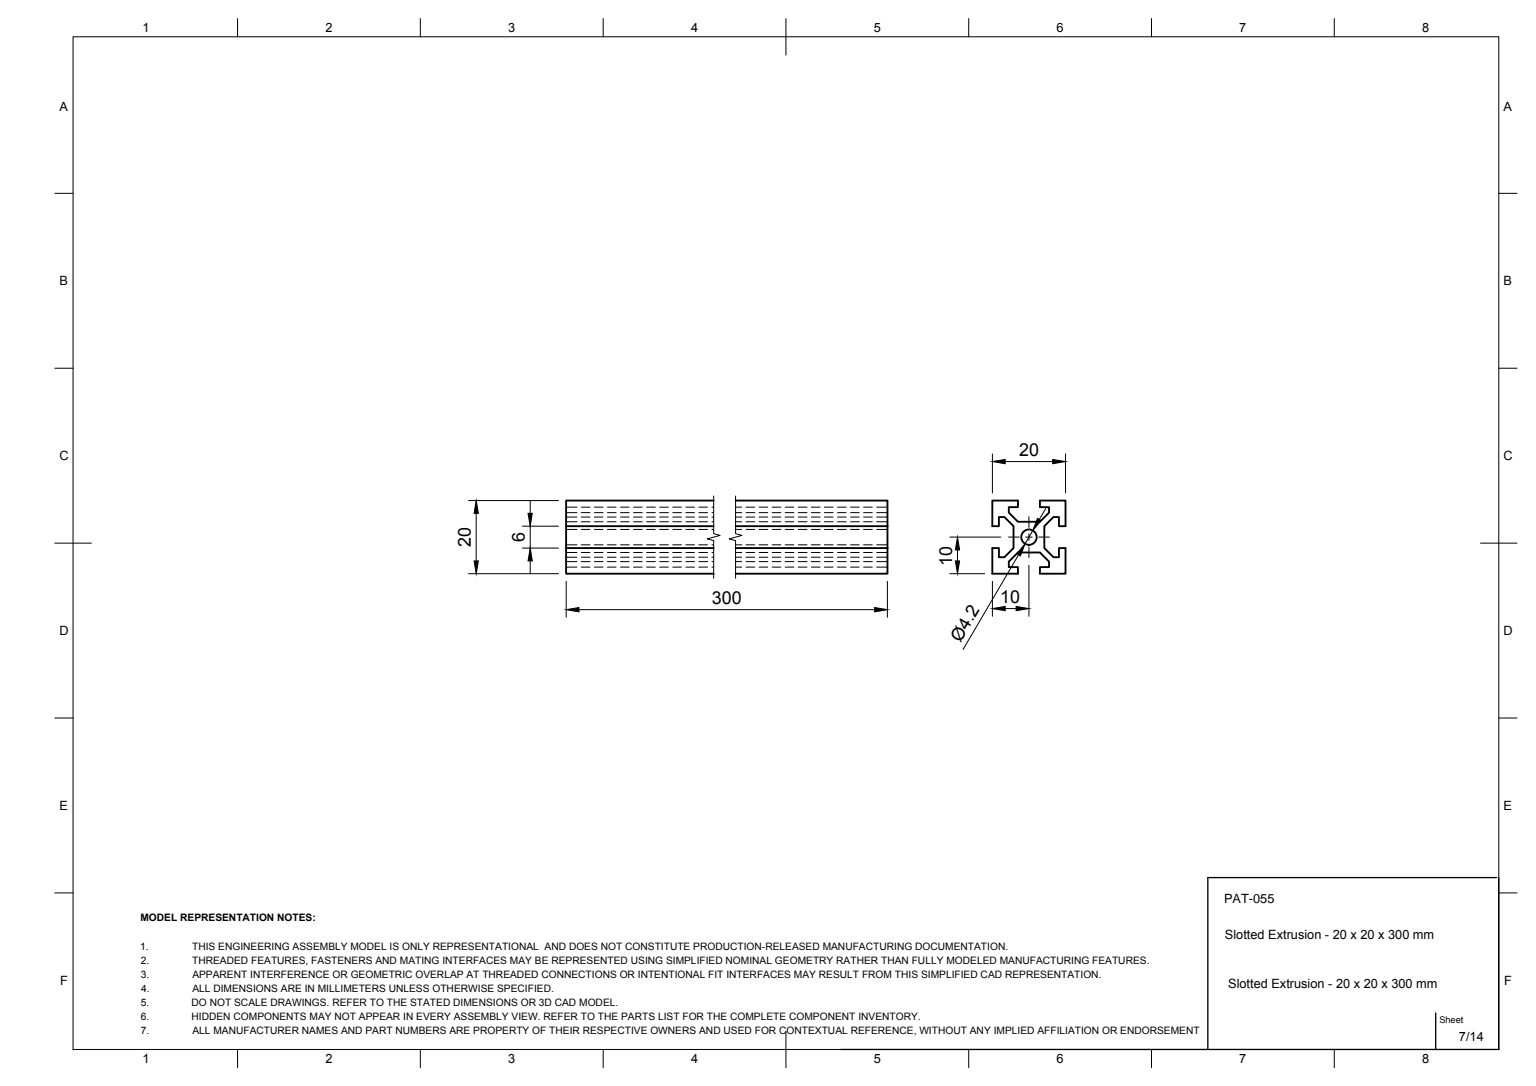
ISO-10303-21;
HEADER;
/* Generated by software containing ST-Developer
 * from STEP Tools, Inc. (www.steptools.com) 
 */

FILE_DESCRIPTION(
/* description */ ('Hinged panel with latch'),
/* implementation_level */ '2;1');

FILE_NAME(
/* name */ 'Slotted Extrusion - 20 x 20 x 300 mm.step',
/* time_stamp */ '2026-10-27T20:36:01-07:00',
/* author */ (''),
/* organization */ (''),
/* preprocessor_version */ 'ST-DEVELOPER v20.2',
/* originating_system */ 'Autodesk Translation Framework v15.17.0.0',
/* authorisation */ '');

FILE_SCHEMA (('AUTOMOTIVE_DESIGN { 1 0 10303 214 3 1 1 }'));
ENDSEC;

DATA;
#10=MECHANICAL_DESIGN_GEOMETRIC_PRESENTATION_REPRESENTATION('',(#297),#6743);
#265=SHAPE_REPRESENTATION_RELATIONSHIP('SRR','None',#6840,#281);
#281=ADVANCED_BREP_SHAPE_REPRESENTATION('',(#313),#6726);
#297=STYLED_ITEM('',(#7017),#313);
#313=MANIFOLD_SOLID_BREP('Body1',#3799);
#329=FACE_BOUND('',#787,.T.);
#330=FACE_BOUND('',#789,.T.);
#378=PLANE('',#4010);
#379=PLANE('',#4011);
#380=PLANE('',#4012);
#381=PLANE('',#4013);
#382=PLANE('',#4014);
#383=PLANE('',#4015);
#384=PLANE('',#4016);
#385=PLANE('',#4017);
#386=PLANE('',#4018);
#387=PLANE('',#4019);
#388=PLANE('',#4020);
#389=PLANE('',#4021);
#390=PLANE('',#4022);
#391=PLANE('',#4023);
#392=PLANE('',#4024);
#393=PLANE('',#4025);
#394=PLANE('',#4026);
#395=PLANE('',#4027);
#396=PLANE('',#4028);
#397=PLANE('',#4029);
#398=PLANE('',#4030);
#399=PLANE('',#4031);
#400=PLANE('',#4032);
#401=PLANE('',#4033);
#402=PLANE('',#4034);
#403=PLANE('',#4035);
#404=PLANE('',#4036);
#405=PLANE('',#4037);
#406=PLANE('',#4038);
#407=PLANE('',#4039);
#408=PLANE('',#4040);
#409=PLANE('',#4041);
#410=PLANE('',#4042);
#411=PLANE('',#4043);
#412=PLANE('',#4044);
#413=PLANE('',#4045);
#414=PLANE('',#4049);
#415=PLANE('',#4050);
#416=PLANE('',#4051);
#417=PLANE('',#4052);
#418=PLANE('',#4053);
#419=PLANE('',#4054);
#420=PLANE('',#4055);
#421=PLANE('',#4056);
#422=PLANE('',#4057);
#423=PLANE('',#4058);
#531=FACE_OUTER_BOUND('',#741,.T.);
#532=FACE_OUTER_BOUND('',#742,.T.);
#533=FACE_OUTER_BOUND('',#743,.T.);
#534=FACE_OUTER_BOUND('',#744,.T.);
#535=FACE_OUTER_BOUND('',#745,.T.);
#536=FACE_OUTER_BOUND('',#746,.T.);
#537=FACE_OUTER_BOUND('',#747,.T.);
#538=FACE_OUTER_BOUND('',#748,.T.);
#539=FACE_OUTER_BOUND('',#749,.T.);
#540=FACE_OUTER_BOUND('',#750,.T.);
#541=FACE_OUTER_BOUND('',#751,.T.);
#542=FACE_OUTER_BOUND('',#752,.T.);
#543=FACE_OUTER_BOUND('',#753,.T.);
#544=FACE_OUTER_BOUND('',#754,.T.);
#545=FACE_OUTER_BOUND('',#755,.T.);
#546=FACE_OUTER_BOUND('',#756,.T.);
#547=FACE_OUTER_BOUND('',#757,.T.);
#548=FACE_OUTER_BOUND('',#758,.T.);
#549=FACE_OUTER_BOUND('',#759,.T.);
#550=FACE_OUTER_BOUND('',#760,.T.);
#551=FACE_OUTER_BOUND('',#761,.T.);
#552=FACE_OUTER_BOUND('',#762,.T.);
#553=FACE_OUTER_BOUND('',#763,.T.);
#554=FACE_OUTER_BOUND('',#764,.T.);
#555=FACE_OUTER_BOUND('',#765,.T.);
#556=FACE_OUTER_BOUND('',#766,.T.);
#557=FACE_OUTER_BOUND('',#767,.T.);
#558=FACE_OUTER_BOUND('',#768,.T.);
#559=FACE_OUTER_BOUND('',#769,.T.);
#560=FACE_OUTER_BOUND('',#770,.T.);
#561=FACE_OUTER_BOUND('',#771,.T.);
#562=FACE_OUTER_BOUND('',#772,.T.);
#563=FACE_OUTER_BOUND('',#773,.T.);
#564=FACE_OUTER_BOUND('',#774,.T.);
#565=FACE_OUTER_BOUND('',#775,.T.);
#566=FACE_OUTER_BOUND('',#776,.T.);
#567=FACE_OUTER_BOUND('',#777,.T.);
#568=FACE_OUTER_BOUND('',#778,.T.);
#569=FACE_OUTER_BOUND('',#779,.T.);
#570=FACE_OUTER_BOUND('',#780,.T.);
#571=FACE_OUTER_BOUND('',#781,.T.);
#572=FACE_OUTER_BOUND('',#782,.T.);
#573=FACE_OUTER_BOUND('',#783,.T.);
#574=FACE_OUTER_BOUND('',#784,.T.);
#575=FACE_OUTER_BOUND('',#785,.T.);
#576=FACE_OUTER_BOUND('',#786,.T.);
#577=FACE_OUTER_BOUND('',#788,.T.);
#741=EDGE_LOOP('',(#2626,#2627,#2628,#2629));
#742=EDGE_LOOP('',(#2630,#2631,#2632,#2633));
#743=EDGE_LOOP('',(#2634,#2635,#2636,#2637));
#744=EDGE_LOOP('',(#2638,#2639,#2640,#2641));
#745=EDGE_LOOP('',(#2642,#2643,#2644,#2645));
#746=EDGE_LOOP('',(#2646,#2647,#2648,#2649));
#747=EDGE_LOOP('',(#2650,#2651,#2652,#2653));
#748=EDGE_LOOP('',(#2654,#2655,#2656,#2657));
#749=EDGE_LOOP('',(#2658,#2659,#2660,#2661));
#750=EDGE_LOOP('',(#2662,#2663,#2664,#2665));
#751=EDGE_LOOP('',(#2666,#2667,#2668,#2669));
#752=EDGE_LOOP('',(#2670,#2671,#2672,#2673));
#753=EDGE_LOOP('',(#2674,#2675,#2676,#2677));
#754=EDGE_LOOP('',(#2678,#2679,#2680,#2681));
#755=EDGE_LOOP('',(#2682,#2683,#2684,#2685));
#756=EDGE_LOOP('',(#2686,#2687,#2688,#2689));
#757=EDGE_LOOP('',(#2690,#2691,#2692,#2693));
#758=EDGE_LOOP('',(#2694,#2695,#2696,#2697));
#759=EDGE_LOOP('',(#2698,#2699,#2700,#2701));
#760=EDGE_LOOP('',(#2702,#2703,#2704,#2705));
#761=EDGE_LOOP('',(#2706,#2707,#2708,#2709));
#762=EDGE_LOOP('',(#2710,#2711,#2712,#2713));
#763=EDGE_LOOP('',(#2714,#2715,#2716,#2717));
#764=EDGE_LOOP('',(#2718,#2719,#2720,#2721));
#765=EDGE_LOOP('',(#2722,#2723,#2724,#2725));
#766=EDGE_LOOP('',(#2726,#2727,#2728,#2729));
#767=EDGE_LOOP('',(#2730,#2731,#2732,#2733));
#768=EDGE_LOOP('',(#2734,#2735,#2736,#2737));
#769=EDGE_LOOP('',(#2738,#2739,#2740,#2741));
#770=EDGE_LOOP('',(#2742,#2743,#2744,#2745));
#771=EDGE_LOOP('',(#2746,#2747,#2748,#2749));
#772=EDGE_LOOP('',(#2750,#2751,#2752,#2753));
#773=EDGE_LOOP('',(#2754,#2755,#2756,#2757));
#774=EDGE_LOOP('',(#2758,#2759,#2760,#2761));
#775=EDGE_LOOP('',(#2762,#2763,#2764,#2765));
#776=EDGE_LOOP('',(#2766,#2767,#2768,#2769));
#777=EDGE_LOOP('',(#2770,#2771,#2772,#2773));
#778=EDGE_LOOP('',(#2774,#2775,#2776,#2777));
#779=EDGE_LOOP('',(#2778,#2779,#2780,#2781));
#780=EDGE_LOOP('',(#2782,#2783,#2784,#2785));
#781=EDGE_LOOP('',(#2786,#2787,#2788,#2789));
#782=EDGE_LOOP('',(#2790,#2791,#2792,#2793));
#783=EDGE_LOOP('',(#2794,#2795,#2796,#2797));
#784=EDGE_LOOP('',(#2798,#2799,#2800,#2801));
#785=EDGE_LOOP('',(#2802,#2803,#2804,#2805));
#786=EDGE_LOOP('',(#2806,#2807,#2808,#2809,#2810,#2811,#2812,#2813,#2814,
#2815,#2816,#2817,#2818,#2819,#2820,#2821,#2822,#2823,#2824,#2825,#2826,
#2827,#2828,#2829,#2830,#2831,#2832,#2833,#2834,#2835,#2836,#2837,#2838,
#2839,#2840,#2841,#2842,#2843,#2844,#2845,#2846,#2847,#2848,#2849));
#787=EDGE_LOOP('',(#2850));
#788=EDGE_LOOP('',(#2851,#2852,#2853,#2854,#2855,#2856,#2857,#2858,#2859,
#2860,#2861,#2862,#2863,#2864,#2865,#2866,#2867,#2868,#2869,#2870,#2871,
#2872,#2873,#2874,#2875,#2876,#2877,#2878,#2879,#2880,#2881,#2882,#2883,
#2884,#2885,#2886,#2887,#2888,#2889,#2890,#2891,#2892,#2893,#2894));
#789=EDGE_LOOP('',(#2895));
#996=LINE('',#5507,#1354);
#997=LINE('',#5509,#1355);
#998=LINE('',#5511,#1356);
#999=LINE('',#5512,#1357);
#1000=LINE('',#5515,#1358);
#1001=LINE('',#5517,#1359);
#1002=LINE('',#5518,#1360);
#1003=LINE('',#5521,#1361);
#1004=LINE('',#5523,#1362);
#1005=LINE('',#5524,#1363);
#1006=LINE('',#5527,#1364);
#1007=LINE('',#5529,#1365);
#1008=LINE('',#5530,#1366);
#1009=LINE('',#5533,#1367);
#1010=LINE('',#5535,#1368);
#1011=LINE('',#5536,#1369);
#1012=LINE('',#5539,#1370);
#1013=LINE('',#5541,#1371);
#1014=LINE('',#5542,#1372);
#1015=LINE('',#5545,#1373);
#1016=LINE('',#5547,#1374);
#1017=LINE('',#5548,#1375);
#1018=LINE('',#5551,#1376);
#1019=LINE('',#5553,#1377);
#1020=LINE('',#5554,#1378);
#1021=LINE('',#5557,#1379);
#1022=LINE('',#5559,#1380);
#1023=LINE('',#5560,#1381);
#1024=LINE('',#5564,#1382);
#1025=LINE('',#5566,#1383);
#1026=LINE('',#5568,#1384);
#1027=LINE('',#5569,#1385);
#1028=LINE('',#5572,#1386);
#1029=LINE('',#5574,#1387);
#1030=LINE('',#5575,#1388);
#1031=LINE('',#5578,#1389);
#1032=LINE('',#5580,#1390);
#1033=LINE('',#5581,#1391);
#1034=LINE('',#5584,#1392);
#1035=LINE('',#5586,#1393);
#1036=LINE('',#5587,#1394);
#1037=LINE('',#5590,#1395);
#1038=LINE('',#5592,#1396);
#1039=LINE('',#5593,#1397);
#1040=LINE('',#5596,#1398);
#1041=LINE('',#5598,#1399);
#1042=LINE('',#5599,#1400);
#1043=LINE('',#5602,#1401);
#1044=LINE('',#5604,#1402);
#1045=LINE('',#5605,#1403);
#1046=LINE('',#5608,#1404);
#1047=LINE('',#5610,#1405);
#1048=LINE('',#5611,#1406);
#1049=LINE('',#5614,#1407);
#1050=LINE('',#5616,#1408);
#1051=LINE('',#5617,#1409);
#1052=LINE('',#5621,#1410);
#1053=LINE('',#5623,#1411);
#1054=LINE('',#5625,#1412);
#1055=LINE('',#5626,#1413);
#1056=LINE('',#5629,#1414);
#1057=LINE('',#5631,#1415);
#1058=LINE('',#5632,#1416);
#1059=LINE('',#5635,#1417);
#1060=LINE('',#5637,#1418);
#1061=LINE('',#5638,#1419);
#1062=LINE('',#5641,#1420);
#1063=LINE('',#5643,#1421);
#1064=LINE('',#5644,#1422);
#1065=LINE('',#5647,#1423);
#1066=LINE('',#5649,#1424);
#1067=LINE('',#5650,#1425);
#1068=LINE('',#5653,#1426);
#1069=LINE('',#5655,#1427);
#1070=LINE('',#5656,#1428);
#1071=LINE('',#5659,#1429);
#1072=LINE('',#5661,#1430);
#1073=LINE('',#5662,#1431);
#1074=LINE('',#5665,#1432);
#1075=LINE('',#5667,#1433);
#1076=LINE('',#5668,#1434);
#1077=LINE('',#5671,#1435);
#1078=LINE('',#5673,#1436);
#1079=LINE('',#5674,#1437);
#1080=LINE('',#5678,#1438);
#1081=LINE('',#5680,#1439);
#1082=LINE('',#5682,#1440);
#1083=LINE('',#5683,#1441);
#1084=LINE('',#5686,#1442);
#1085=LINE('',#5688,#1443);
#1086=LINE('',#5689,#1444);
#1087=LINE('',#5692,#1445);
#1088=LINE('',#5694,#1446);
#1089=LINE('',#5695,#1447);
#1090=LINE('',#5698,#1448);
#1091=LINE('',#5700,#1449);
#1092=LINE('',#5701,#1450);
#1093=LINE('',#5704,#1451);
#1094=LINE('',#5706,#1452);
#1095=LINE('',#5707,#1453);
#1096=LINE('',#5710,#1454);
#1097=LINE('',#5712,#1455);
#1098=LINE('',#5713,#1456);
#1099=LINE('',#5716,#1457);
#1100=LINE('',#5718,#1458);
#1101=LINE('',#5719,#1459);
#1102=LINE('',#5722,#1460);
#1103=LINE('',#5724,#1461);
#1104=LINE('',#5725,#1462);
#1105=LINE('',#5728,#1463);
#1106=LINE('',#5730,#1464);
#1107=LINE('',#5731,#1465);
#1108=LINE('',#5736,#1466);
#1109=LINE('',#5740,#1467);
#1110=LINE('',#5742,#1468);
#1111=LINE('',#5743,#1469);
#1112=LINE('',#5746,#1470);
#1113=LINE('',#5748,#1471);
#1114=LINE('',#5749,#1472);
#1115=LINE('',#5751,#1473);
#1116=LINE('',#5752,#1474);
#1117=LINE('',#5755,#1475);
#1118=LINE('',#5757,#1476);
#1119=LINE('',#5758,#1477);
#1120=LINE('',#5760,#1478);
#1121=LINE('',#5761,#1479);
#1122=LINE('',#5764,#1480);
#1123=LINE('',#5766,#1481);
#1124=LINE('',#5767,#1482);
#1125=LINE('',#5769,#1483);
#1126=LINE('',#5770,#1484);
#1127=LINE('',#5772,#1485);
#1128=LINE('',#5773,#1486);
#1354=VECTOR('',#4412,1.);
#1355=VECTOR('',#4413,1.);
#1356=VECTOR('',#4414,1.);
#1357=VECTOR('',#4415,1.);
#1358=VECTOR('',#4418,1.);
#1359=VECTOR('',#4419,1.);
#1360=VECTOR('',#4420,1.);
#1361=VECTOR('',#4423,1.);
#1362=VECTOR('',#4424,1.);
#1363=VECTOR('',#4425,1.);
#1364=VECTOR('',#4428,1.);
#1365=VECTOR('',#4429,1.);
#1366=VECTOR('',#4430,1.);
#1367=VECTOR('',#4433,1.);
#1368=VECTOR('',#4434,1.);
#1369=VECTOR('',#4435,1.);
#1370=VECTOR('',#4438,1.);
#1371=VECTOR('',#4439,1.);
#1372=VECTOR('',#4440,1.);
#1373=VECTOR('',#4443,1.);
#1374=VECTOR('',#4444,1.);
#1375=VECTOR('',#4445,1.);
#1376=VECTOR('',#4448,1.);
#1377=VECTOR('',#4449,1.);
#1378=VECTOR('',#4450,1.);
#1379=VECTOR('',#4453,1.);
#1380=VECTOR('',#4454,1.);
#1381=VECTOR('',#4455,1.);
#1382=VECTOR('',#4458,1.);
#1383=VECTOR('',#4459,1.);
#1384=VECTOR('',#4460,1.);
#1385=VECTOR('',#4461,1.);
#1386=VECTOR('',#4464,1.);
#1387=VECTOR('',#4465,1.);
#1388=VECTOR('',#4466,1.);
#1389=VECTOR('',#4469,1.);
#1390=VECTOR('',#4470,1.);
#1391=VECTOR('',#4471,1.);
#1392=VECTOR('',#4474,1.);
#1393=VECTOR('',#4475,1.);
#1394=VECTOR('',#4476,1.);
#1395=VECTOR('',#4479,1.);
#1396=VECTOR('',#4480,1.);
#1397=VECTOR('',#4481,1.);
#1398=VECTOR('',#4484,1.);
#1399=VECTOR('',#4485,1.);
#1400=VECTOR('',#4486,1.);
#1401=VECTOR('',#4489,1.);
#1402=VECTOR('',#4490,1.);
#1403=VECTOR('',#4491,1.);
#1404=VECTOR('',#4494,1.);
#1405=VECTOR('',#4495,1.);
#1406=VECTOR('',#4496,1.);
#1407=VECTOR('',#4499,1.);
#1408=VECTOR('',#4500,1.);
#1409=VECTOR('',#4501,1.);
#1410=VECTOR('',#4504,1.);
#1411=VECTOR('',#4505,1.);
#1412=VECTOR('',#4506,1.);
#1413=VECTOR('',#4507,1.);
#1414=VECTOR('',#4510,1.);
#1415=VECTOR('',#4511,1.);
#1416=VECTOR('',#4512,1.);
#1417=VECTOR('',#4515,1.);
#1418=VECTOR('',#4516,1.);
#1419=VECTOR('',#4517,1.);
#1420=VECTOR('',#4520,1.);
#1421=VECTOR('',#4521,1.);
#1422=VECTOR('',#4522,1.);
#1423=VECTOR('',#4525,1.);
#1424=VECTOR('',#4526,1.);
#1425=VECTOR('',#4527,1.);
#1426=VECTOR('',#4530,1.);
#1427=VECTOR('',#4531,1.);
#1428=VECTOR('',#4532,1.);
#1429=VECTOR('',#4535,1.);
#1430=VECTOR('',#4536,1.);
#1431=VECTOR('',#4537,1.);
#1432=VECTOR('',#4540,1.);
#1433=VECTOR('',#4541,1.);
#1434=VECTOR('',#4542,1.);
#1435=VECTOR('',#4545,1.);
#1436=VECTOR('',#4546,1.);
#1437=VECTOR('',#4547,1.);
#1438=VECTOR('',#4550,1.);
#1439=VECTOR('',#4551,1.);
#1440=VECTOR('',#4552,1.);
#1441=VECTOR('',#4553,1.);
#1442=VECTOR('',#4556,1.);
#1443=VECTOR('',#4557,1.);
#1444=VECTOR('',#4558,1.);
#1445=VECTOR('',#4561,1.);
#1446=VECTOR('',#4562,1.);
#1447=VECTOR('',#4563,1.);
#1448=VECTOR('',#4566,1.);
#1449=VECTOR('',#4567,1.);
#1450=VECTOR('',#4568,1.);
#1451=VECTOR('',#4571,1.);
#1452=VECTOR('',#4572,1.);
#1453=VECTOR('',#4573,1.);
#1454=VECTOR('',#4576,1.);
#1455=VECTOR('',#4577,1.);
#1456=VECTOR('',#4578,1.);
#1457=VECTOR('',#4581,1.);
#1458=VECTOR('',#4582,1.);
#1459=VECTOR('',#4583,1.);
#1460=VECTOR('',#4586,1.);
#1461=VECTOR('',#4587,1.);
#1462=VECTOR('',#4588,1.);
#1463=VECTOR('',#4591,1.);
#1464=VECTOR('',#4592,1.);
#1465=VECTOR('',#4593,1.);
#1466=VECTOR('',#4598,0.21);
#1467=VECTOR('',#4603,1.);
#1468=VECTOR('',#4604,1.);
#1469=VECTOR('',#4605,1.);
#1470=VECTOR('',#4608,1.);
#1471=VECTOR('',#4609,1.);
#1472=VECTOR('',#4610,1.);
#1473=VECTOR('',#4613,1.);
#1474=VECTOR('',#4614,1.);
#1475=VECTOR('',#4617,1.);
#1476=VECTOR('',#4618,1.);
#1477=VECTOR('',#4619,1.);
#1478=VECTOR('',#4622,1.);
#1479=VECTOR('',#4623,1.);
#1480=VECTOR('',#4626,1.);
#1481=VECTOR('',#4627,1.);
#1482=VECTOR('',#4628,1.);
#1483=VECTOR('',#4631,1.);
#1484=VECTOR('',#4632,1.);
#1485=VECTOR('',#4635,1.);
#1486=VECTOR('',#4636,1.);
#1702=CIRCLE('',#4047,0.21);
#1703=CIRCLE('',#4048,0.21);
#1803=VERTEX_POINT('',#5505);
#1804=VERTEX_POINT('',#5506);
#1805=VERTEX_POINT('',#5508);
#1806=VERTEX_POINT('',#5510);
#1807=VERTEX_POINT('',#5514);
#1808=VERTEX_POINT('',#5516);
#1809=VERTEX_POINT('',#5520);
#1810=VERTEX_POINT('',#5522);
#1811=VERTEX_POINT('',#5526);
#1812=VERTEX_POINT('',#5528);
#1813=VERTEX_POINT('',#5532);
#1814=VERTEX_POINT('',#5534);
#1815=VERTEX_POINT('',#5538);
#1816=VERTEX_POINT('',#5540);
#1817=VERTEX_POINT('',#5544);
#1818=VERTEX_POINT('',#5546);
#1819=VERTEX_POINT('',#5550);
#1820=VERTEX_POINT('',#5552);
#1821=VERTEX_POINT('',#5556);
#1822=VERTEX_POINT('',#5558);
#1823=VERTEX_POINT('',#5562);
#1824=VERTEX_POINT('',#5563);
#1825=VERTEX_POINT('',#5565);
#1826=VERTEX_POINT('',#5567);
#1827=VERTEX_POINT('',#5571);
#1828=VERTEX_POINT('',#5573);
#1829=VERTEX_POINT('',#5577);
#1830=VERTEX_POINT('',#5579);
#1831=VERTEX_POINT('',#5583);
#1832=VERTEX_POINT('',#5585);
#1833=VERTEX_POINT('',#5589);
#1834=VERTEX_POINT('',#5591);
#1835=VERTEX_POINT('',#5595);
#1836=VERTEX_POINT('',#5597);
#1837=VERTEX_POINT('',#5601);
#1838=VERTEX_POINT('',#5603);
#1839=VERTEX_POINT('',#5607);
#1840=VERTEX_POINT('',#5609);
#1841=VERTEX_POINT('',#5613);
#1842=VERTEX_POINT('',#5615);
#1843=VERTEX_POINT('',#5619);
#1844=VERTEX_POINT('',#5620);
#1845=VERTEX_POINT('',#5622);
#1846=VERTEX_POINT('',#5624);
#1847=VERTEX_POINT('',#5628);
#1848=VERTEX_POINT('',#5630);
#1849=VERTEX_POINT('',#5634);
#1850=VERTEX_POINT('',#5636);
#1851=VERTEX_POINT('',#5640);
#1852=VERTEX_POINT('',#5642);
#1853=VERTEX_POINT('',#5646);
#1854=VERTEX_POINT('',#5648);
#1855=VERTEX_POINT('',#5652);
#1856=VERTEX_POINT('',#5654);
#1857=VERTEX_POINT('',#5658);
#1858=VERTEX_POINT('',#5660);
#1859=VERTEX_POINT('',#5664);
#1860=VERTEX_POINT('',#5666);
#1861=VERTEX_POINT('',#5670);
#1862=VERTEX_POINT('',#5672);
#1863=VERTEX_POINT('',#5676);
#1864=VERTEX_POINT('',#5677);
#1865=VERTEX_POINT('',#5679);
#1866=VERTEX_POINT('',#5681);
#1867=VERTEX_POINT('',#5685);
#1868=VERTEX_POINT('',#5687);
#1869=VERTEX_POINT('',#5691);
#1870=VERTEX_POINT('',#5693);
#1871=VERTEX_POINT('',#5697);
#1872=VERTEX_POINT('',#5699);
#1873=VERTEX_POINT('',#5703);
#1874=VERTEX_POINT('',#5705);
#1875=VERTEX_POINT('',#5709);
#1876=VERTEX_POINT('',#5711);
#1877=VERTEX_POINT('',#5715);
#1878=VERTEX_POINT('',#5717);
#1879=VERTEX_POINT('',#5721);
#1880=VERTEX_POINT('',#5723);
#1881=VERTEX_POINT('',#5727);
#1882=VERTEX_POINT('',#5729);
#1883=VERTEX_POINT('',#5733);
#1884=VERTEX_POINT('',#5735);
#1885=VERTEX_POINT('',#5739);
#1886=VERTEX_POINT('',#5741);
#1887=VERTEX_POINT('',#5745);
#1888=VERTEX_POINT('',#5747);
#1889=VERTEX_POINT('',#5754);
#1890=VERTEX_POINT('',#5756);
#1891=VERTEX_POINT('',#5763);
#1892=VERTEX_POINT('',#5765);
#2125=EDGE_CURVE('',#1803,#1804,#996,.T.);
#2126=EDGE_CURVE('',#1803,#1805,#997,.T.);
#2127=EDGE_CURVE('',#1806,#1805,#998,.T.);
#2128=EDGE_CURVE('',#1804,#1806,#999,.T.);
#2129=EDGE_CURVE('',#1807,#1803,#1000,.T.);
#2130=EDGE_CURVE('',#1807,#1808,#1001,.T.);
#2131=EDGE_CURVE('',#1805,#1808,#1002,.T.);
#2132=EDGE_CURVE('',#1809,#1807,#1003,.T.);
#2133=EDGE_CURVE('',#1809,#1810,#1004,.T.);
#2134=EDGE_CURVE('',#1808,#1810,#1005,.T.);
#2135=EDGE_CURVE('',#1811,#1809,#1006,.T.);
#2136=EDGE_CURVE('',#1811,#1812,#1007,.T.);
#2137=EDGE_CURVE('',#1810,#1812,#1008,.T.);
#2138=EDGE_CURVE('',#1813,#1811,#1009,.T.);
#2139=EDGE_CURVE('',#1813,#1814,#1010,.T.);
#2140=EDGE_CURVE('',#1812,#1814,#1011,.T.);
#2141=EDGE_CURVE('',#1815,#1813,#1012,.T.);
#2142=EDGE_CURVE('',#1815,#1816,#1013,.T.);
#2143=EDGE_CURVE('',#1814,#1816,#1014,.T.);
#2144=EDGE_CURVE('',#1817,#1815,#1015,.T.);
#2145=EDGE_CURVE('',#1817,#1818,#1016,.T.);
#2146=EDGE_CURVE('',#1816,#1818,#1017,.T.);
#2147=EDGE_CURVE('',#1819,#1817,#1018,.T.);
#2148=EDGE_CURVE('',#1819,#1820,#1019,.T.);
#2149=EDGE_CURVE('',#1818,#1820,#1020,.T.);
#2150=EDGE_CURVE('',#1821,#1819,#1021,.T.);
#2151=EDGE_CURVE('',#1822,#1821,#1022,.T.);
#2152=EDGE_CURVE('',#1820,#1822,#1023,.T.);
#2153=EDGE_CURVE('',#1823,#1824,#1024,.T.);
#2154=EDGE_CURVE('',#1823,#1825,#1025,.T.);
#2155=EDGE_CURVE('',#1826,#1825,#1026,.T.);
#2156=EDGE_CURVE('',#1824,#1826,#1027,.T.);
#2157=EDGE_CURVE('',#1827,#1823,#1028,.T.);
#2158=EDGE_CURVE('',#1827,#1828,#1029,.T.);
#2159=EDGE_CURVE('',#1825,#1828,#1030,.T.);
#2160=EDGE_CURVE('',#1829,#1827,#1031,.T.);
#2161=EDGE_CURVE('',#1829,#1830,#1032,.T.);
#2162=EDGE_CURVE('',#1828,#1830,#1033,.T.);
#2163=EDGE_CURVE('',#1831,#1829,#1034,.T.);
#2164=EDGE_CURVE('',#1831,#1832,#1035,.T.);
#2165=EDGE_CURVE('',#1830,#1832,#1036,.T.);
#2166=EDGE_CURVE('',#1833,#1831,#1037,.T.);
#2167=EDGE_CURVE('',#1833,#1834,#1038,.T.);
#2168=EDGE_CURVE('',#1832,#1834,#1039,.T.);
#2169=EDGE_CURVE('',#1835,#1833,#1040,.T.);
#2170=EDGE_CURVE('',#1835,#1836,#1041,.T.);
#2171=EDGE_CURVE('',#1834,#1836,#1042,.T.);
#2172=EDGE_CURVE('',#1837,#1835,#1043,.T.);
#2173=EDGE_CURVE('',#1837,#1838,#1044,.T.);
#2174=EDGE_CURVE('',#1836,#1838,#1045,.T.);
#2175=EDGE_CURVE('',#1839,#1837,#1046,.T.);
#2176=EDGE_CURVE('',#1839,#1840,#1047,.T.);
#2177=EDGE_CURVE('',#1838,#1840,#1048,.T.);
#2178=EDGE_CURVE('',#1841,#1839,#1049,.T.);
#2179=EDGE_CURVE('',#1842,#1841,#1050,.T.);
#2180=EDGE_CURVE('',#1840,#1842,#1051,.T.);
#2181=EDGE_CURVE('',#1843,#1844,#1052,.T.);
#2182=EDGE_CURVE('',#1843,#1845,#1053,.T.);
#2183=EDGE_CURVE('',#1846,#1845,#1054,.T.);
#2184=EDGE_CURVE('',#1844,#1846,#1055,.T.);
#2185=EDGE_CURVE('',#1847,#1843,#1056,.T.);
#2186=EDGE_CURVE('',#1847,#1848,#1057,.T.);
#2187=EDGE_CURVE('',#1845,#1848,#1058,.T.);
#2188=EDGE_CURVE('',#1849,#1847,#1059,.T.);
#2189=EDGE_CURVE('',#1849,#1850,#1060,.T.);
#2190=EDGE_CURVE('',#1848,#1850,#1061,.T.);
#2191=EDGE_CURVE('',#1851,#1849,#1062,.T.);
#2192=EDGE_CURVE('',#1851,#1852,#1063,.T.);
#2193=EDGE_CURVE('',#1850,#1852,#1064,.T.);
#2194=EDGE_CURVE('',#1853,#1851,#1065,.T.);
#2195=EDGE_CURVE('',#1853,#1854,#1066,.T.);
#2196=EDGE_CURVE('',#1852,#1854,#1067,.T.);
#2197=EDGE_CURVE('',#1855,#1853,#1068,.T.);
#2198=EDGE_CURVE('',#1855,#1856,#1069,.T.);
#2199=EDGE_CURVE('',#1854,#1856,#1070,.T.);
#2200=EDGE_CURVE('',#1857,#1855,#1071,.T.);
#2201=EDGE_CURVE('',#1857,#1858,#1072,.T.);
#2202=EDGE_CURVE('',#1856,#1858,#1073,.T.);
#2203=EDGE_CURVE('',#1859,#1857,#1074,.T.);
#2204=EDGE_CURVE('',#1859,#1860,#1075,.T.);
#2205=EDGE_CURVE('',#1858,#1860,#1076,.T.);
#2206=EDGE_CURVE('',#1861,#1859,#1077,.T.);
#2207=EDGE_CURVE('',#1862,#1861,#1078,.T.);
#2208=EDGE_CURVE('',#1860,#1862,#1079,.T.);
#2209=EDGE_CURVE('',#1863,#1864,#1080,.T.);
#2210=EDGE_CURVE('',#1863,#1865,#1081,.T.);
#2211=EDGE_CURVE('',#1866,#1865,#1082,.T.);
#2212=EDGE_CURVE('',#1864,#1866,#1083,.T.);
#2213=EDGE_CURVE('',#1867,#1863,#1084,.T.);
#2214=EDGE_CURVE('',#1867,#1868,#1085,.T.);
#2215=EDGE_CURVE('',#1865,#1868,#1086,.T.);
#2216=EDGE_CURVE('',#1869,#1867,#1087,.T.);
#2217=EDGE_CURVE('',#1869,#1870,#1088,.T.);
#2218=EDGE_CURVE('',#1868,#1870,#1089,.T.);
#2219=EDGE_CURVE('',#1871,#1869,#1090,.T.);
#2220=EDGE_CURVE('',#1871,#1872,#1091,.T.);
#2221=EDGE_CURVE('',#1870,#1872,#1092,.T.);
#2222=EDGE_CURVE('',#1873,#1871,#1093,.T.);
#2223=EDGE_CURVE('',#1873,#1874,#1094,.T.);
#2224=EDGE_CURVE('',#1872,#1874,#1095,.T.);
#2225=EDGE_CURVE('',#1875,#1873,#1096,.T.);
#2226=EDGE_CURVE('',#1875,#1876,#1097,.T.);
#2227=EDGE_CURVE('',#1874,#1876,#1098,.T.);
#2228=EDGE_CURVE('',#1877,#1875,#1099,.T.);
#2229=EDGE_CURVE('',#1877,#1878,#1100,.T.);
#2230=EDGE_CURVE('',#1876,#1878,#1101,.T.);
#2231=EDGE_CURVE('',#1879,#1877,#1102,.T.);
#2232=EDGE_CURVE('',#1879,#1880,#1103,.T.);
#2233=EDGE_CURVE('',#1878,#1880,#1104,.T.);
#2234=EDGE_CURVE('',#1881,#1879,#1105,.T.);
#2235=EDGE_CURVE('',#1882,#1881,#1106,.T.);
#2236=EDGE_CURVE('',#1880,#1882,#1107,.T.);
#2237=EDGE_CURVE('',#1883,#1883,#1702,.T.);
#2238=EDGE_CURVE('',#1883,#1884,#1108,.T.);
#2239=EDGE_CURVE('',#1884,#1884,#1703,.T.);
#2240=EDGE_CURVE('',#1821,#1885,#1109,.T.);
#2241=EDGE_CURVE('',#1885,#1886,#1110,.T.);
#2242=EDGE_CURVE('',#1822,#1886,#1111,.T.);
#2243=EDGE_CURVE('',#1887,#1806,#1112,.T.);
#2244=EDGE_CURVE('',#1888,#1887,#1113,.T.);
#2245=EDGE_CURVE('',#1888,#1804,#1114,.T.);
#2246=EDGE_CURVE('',#1841,#1888,#1115,.T.);
#2247=EDGE_CURVE('',#1842,#1887,#1116,.T.);
#2248=EDGE_CURVE('',#1889,#1826,#1117,.T.);
#2249=EDGE_CURVE('',#1890,#1889,#1118,.T.);
#2250=EDGE_CURVE('',#1890,#1824,#1119,.T.);
#2251=EDGE_CURVE('',#1861,#1890,#1120,.T.);
#2252=EDGE_CURVE('',#1862,#1889,#1121,.T.);
#2253=EDGE_CURVE('',#1891,#1846,#1122,.T.);
#2254=EDGE_CURVE('',#1892,#1891,#1123,.T.);
#2255=EDGE_CURVE('',#1892,#1844,#1124,.T.);
#2256=EDGE_CURVE('',#1881,#1892,#1125,.T.);
#2257=EDGE_CURVE('',#1882,#1891,#1126,.T.);
#2258=EDGE_CURVE('',#1886,#1866,#1127,.T.);
#2259=EDGE_CURVE('',#1885,#1864,#1128,.T.);
#2626=ORIENTED_EDGE('',*,*,#2125,.F.);
#2627=ORIENTED_EDGE('',*,*,#2126,.T.);
#2628=ORIENTED_EDGE('',*,*,#2127,.F.);
#2629=ORIENTED_EDGE('',*,*,#2128,.F.);
#2630=ORIENTED_EDGE('',*,*,#2129,.F.);
#2631=ORIENTED_EDGE('',*,*,#2130,.T.);
#2632=ORIENTED_EDGE('',*,*,#2131,.F.);
#2633=ORIENTED_EDGE('',*,*,#2126,.F.);
#2634=ORIENTED_EDGE('',*,*,#2132,.F.);
#2635=ORIENTED_EDGE('',*,*,#2133,.T.);
#2636=ORIENTED_EDGE('',*,*,#2134,.F.);
#2637=ORIENTED_EDGE('',*,*,#2130,.F.);
#2638=ORIENTED_EDGE('',*,*,#2135,.F.);
#2639=ORIENTED_EDGE('',*,*,#2136,.T.);
#2640=ORIENTED_EDGE('',*,*,#2137,.F.);
#2641=ORIENTED_EDGE('',*,*,#2133,.F.);
#2642=ORIENTED_EDGE('',*,*,#2138,.F.);
#2643=ORIENTED_EDGE('',*,*,#2139,.T.);
#2644=ORIENTED_EDGE('',*,*,#2140,.F.);
#2645=ORIENTED_EDGE('',*,*,#2136,.F.);
#2646=ORIENTED_EDGE('',*,*,#2141,.F.);
#2647=ORIENTED_EDGE('',*,*,#2142,.T.);
#2648=ORIENTED_EDGE('',*,*,#2143,.F.);
#2649=ORIENTED_EDGE('',*,*,#2139,.F.);
#2650=ORIENTED_EDGE('',*,*,#2144,.F.);
#2651=ORIENTED_EDGE('',*,*,#2145,.T.);
#2652=ORIENTED_EDGE('',*,*,#2146,.F.);
#2653=ORIENTED_EDGE('',*,*,#2142,.F.);
#2654=ORIENTED_EDGE('',*,*,#2147,.F.);
#2655=ORIENTED_EDGE('',*,*,#2148,.T.);
#2656=ORIENTED_EDGE('',*,*,#2149,.F.);
#2657=ORIENTED_EDGE('',*,*,#2145,.F.);
#2658=ORIENTED_EDGE('',*,*,#2150,.F.);
#2659=ORIENTED_EDGE('',*,*,#2151,.F.);
#2660=ORIENTED_EDGE('',*,*,#2152,.F.);
#2661=ORIENTED_EDGE('',*,*,#2148,.F.);
#2662=ORIENTED_EDGE('',*,*,#2153,.F.);
#2663=ORIENTED_EDGE('',*,*,#2154,.T.);
#2664=ORIENTED_EDGE('',*,*,#2155,.F.);
#2665=ORIENTED_EDGE('',*,*,#2156,.F.);
#2666=ORIENTED_EDGE('',*,*,#2157,.F.);
#2667=ORIENTED_EDGE('',*,*,#2158,.T.);
#2668=ORIENTED_EDGE('',*,*,#2159,.F.);
#2669=ORIENTED_EDGE('',*,*,#2154,.F.);
#2670=ORIENTED_EDGE('',*,*,#2160,.F.);
#2671=ORIENTED_EDGE('',*,*,#2161,.T.);
#2672=ORIENTED_EDGE('',*,*,#2162,.F.);
#2673=ORIENTED_EDGE('',*,*,#2158,.F.);
#2674=ORIENTED_EDGE('',*,*,#2163,.F.);
#2675=ORIENTED_EDGE('',*,*,#2164,.T.);
#2676=ORIENTED_EDGE('',*,*,#2165,.F.);
#2677=ORIENTED_EDGE('',*,*,#2161,.F.);
#2678=ORIENTED_EDGE('',*,*,#2166,.F.);
#2679=ORIENTED_EDGE('',*,*,#2167,.T.);
#2680=ORIENTED_EDGE('',*,*,#2168,.F.);
#2681=ORIENTED_EDGE('',*,*,#2164,.F.);
#2682=ORIENTED_EDGE('',*,*,#2169,.F.);
#2683=ORIENTED_EDGE('',*,*,#2170,.T.);
#2684=ORIENTED_EDGE('',*,*,#2171,.F.);
#2685=ORIENTED_EDGE('',*,*,#2167,.F.);
#2686=ORIENTED_EDGE('',*,*,#2172,.F.);
#2687=ORIENTED_EDGE('',*,*,#2173,.T.);
#2688=ORIENTED_EDGE('',*,*,#2174,.F.);
#2689=ORIENTED_EDGE('',*,*,#2170,.F.);
#2690=ORIENTED_EDGE('',*,*,#2175,.F.);
#2691=ORIENTED_EDGE('',*,*,#2176,.T.);
#2692=ORIENTED_EDGE('',*,*,#2177,.F.);
#2693=ORIENTED_EDGE('',*,*,#2173,.F.);
#2694=ORIENTED_EDGE('',*,*,#2178,.F.);
#2695=ORIENTED_EDGE('',*,*,#2179,.F.);
#2696=ORIENTED_EDGE('',*,*,#2180,.F.);
#2697=ORIENTED_EDGE('',*,*,#2176,.F.);
#2698=ORIENTED_EDGE('',*,*,#2181,.F.);
#2699=ORIENTED_EDGE('',*,*,#2182,.T.);
#2700=ORIENTED_EDGE('',*,*,#2183,.F.);
#2701=ORIENTED_EDGE('',*,*,#2184,.F.);
#2702=ORIENTED_EDGE('',*,*,#2185,.F.);
#2703=ORIENTED_EDGE('',*,*,#2186,.T.);
#2704=ORIENTED_EDGE('',*,*,#2187,.F.);
#2705=ORIENTED_EDGE('',*,*,#2182,.F.);
#2706=ORIENTED_EDGE('',*,*,#2188,.F.);
#2707=ORIENTED_EDGE('',*,*,#2189,.T.);
#2708=ORIENTED_EDGE('',*,*,#2190,.F.);
#2709=ORIENTED_EDGE('',*,*,#2186,.F.);
#2710=ORIENTED_EDGE('',*,*,#2191,.F.);
#2711=ORIENTED_EDGE('',*,*,#2192,.T.);
#2712=ORIENTED_EDGE('',*,*,#2193,.F.);
#2713=ORIENTED_EDGE('',*,*,#2189,.F.);
#2714=ORIENTED_EDGE('',*,*,#2194,.F.);
#2715=ORIENTED_EDGE('',*,*,#2195,.T.);
#2716=ORIENTED_EDGE('',*,*,#2196,.F.);
#2717=ORIENTED_EDGE('',*,*,#2192,.F.);
#2718=ORIENTED_EDGE('',*,*,#2197,.F.);
#2719=ORIENTED_EDGE('',*,*,#2198,.T.);
#2720=ORIENTED_EDGE('',*,*,#2199,.F.);
#2721=ORIENTED_EDGE('',*,*,#2195,.F.);
#2722=ORIENTED_EDGE('',*,*,#2200,.F.);
#2723=ORIENTED_EDGE('',*,*,#2201,.T.);
#2724=ORIENTED_EDGE('',*,*,#2202,.F.);
#2725=ORIENTED_EDGE('',*,*,#2198,.F.);
#2726=ORIENTED_EDGE('',*,*,#2203,.F.);
#2727=ORIENTED_EDGE('',*,*,#2204,.T.);
#2728=ORIENTED_EDGE('',*,*,#2205,.F.);
#2729=ORIENTED_EDGE('',*,*,#2201,.F.);
#2730=ORIENTED_EDGE('',*,*,#2206,.F.);
#2731=ORIENTED_EDGE('',*,*,#2207,.F.);
#2732=ORIENTED_EDGE('',*,*,#2208,.F.);
#2733=ORIENTED_EDGE('',*,*,#2204,.F.);
#2734=ORIENTED_EDGE('',*,*,#2209,.F.);
#2735=ORIENTED_EDGE('',*,*,#2210,.T.);
#2736=ORIENTED_EDGE('',*,*,#2211,.F.);
#2737=ORIENTED_EDGE('',*,*,#2212,.F.);
#2738=ORIENTED_EDGE('',*,*,#2213,.F.);
#2739=ORIENTED_EDGE('',*,*,#2214,.T.);
#2740=ORIENTED_EDGE('',*,*,#2215,.F.);
#2741=ORIENTED_EDGE('',*,*,#2210,.F.);
#2742=ORIENTED_EDGE('',*,*,#2216,.F.);
#2743=ORIENTED_EDGE('',*,*,#2217,.T.);
#2744=ORIENTED_EDGE('',*,*,#2218,.F.);
#2745=ORIENTED_EDGE('',*,*,#2214,.F.);
#2746=ORIENTED_EDGE('',*,*,#2219,.F.);
#2747=ORIENTED_EDGE('',*,*,#2220,.T.);
#2748=ORIENTED_EDGE('',*,*,#2221,.F.);
#2749=ORIENTED_EDGE('',*,*,#2217,.F.);
#2750=ORIENTED_EDGE('',*,*,#2222,.F.);
#2751=ORIENTED_EDGE('',*,*,#2223,.T.);
#2752=ORIENTED_EDGE('',*,*,#2224,.F.);
#2753=ORIENTED_EDGE('',*,*,#2220,.F.);
#2754=ORIENTED_EDGE('',*,*,#2225,.F.);
#2755=ORIENTED_EDGE('',*,*,#2226,.T.);
#2756=ORIENTED_EDGE('',*,*,#2227,.F.);
#2757=ORIENTED_EDGE('',*,*,#2223,.F.);
#2758=ORIENTED_EDGE('',*,*,#2228,.F.);
#2759=ORIENTED_EDGE('',*,*,#2229,.T.);
#2760=ORIENTED_EDGE('',*,*,#2230,.F.);
#2761=ORIENTED_EDGE('',*,*,#2226,.F.);
#2762=ORIENTED_EDGE('',*,*,#2231,.F.);
#2763=ORIENTED_EDGE('',*,*,#2232,.T.);
#2764=ORIENTED_EDGE('',*,*,#2233,.F.);
#2765=ORIENTED_EDGE('',*,*,#2229,.F.);
#2766=ORIENTED_EDGE('',*,*,#2234,.F.);
#2767=ORIENTED_EDGE('',*,*,#2235,.F.);
#2768=ORIENTED_EDGE('',*,*,#2236,.F.);
#2769=ORIENTED_EDGE('',*,*,#2232,.F.);
#2770=ORIENTED_EDGE('',*,*,#2237,.F.);
#2771=ORIENTED_EDGE('',*,*,#2238,.T.);
#2772=ORIENTED_EDGE('',*,*,#2239,.F.);
#2773=ORIENTED_EDGE('',*,*,#2238,.F.);
#2774=ORIENTED_EDGE('',*,*,#2151,.T.);
#2775=ORIENTED_EDGE('',*,*,#2240,.T.);
#2776=ORIENTED_EDGE('',*,*,#2241,.T.);
#2777=ORIENTED_EDGE('',*,*,#2242,.F.);
#2778=ORIENTED_EDGE('',*,*,#2128,.T.);
#2779=ORIENTED_EDGE('',*,*,#2243,.F.);
#2780=ORIENTED_EDGE('',*,*,#2244,.F.);
#2781=ORIENTED_EDGE('',*,*,#2245,.T.);
#2782=ORIENTED_EDGE('',*,*,#2179,.T.);
#2783=ORIENTED_EDGE('',*,*,#2246,.T.);
#2784=ORIENTED_EDGE('',*,*,#2244,.T.);
#2785=ORIENTED_EDGE('',*,*,#2247,.F.);
#2786=ORIENTED_EDGE('',*,*,#2156,.T.);
#2787=ORIENTED_EDGE('',*,*,#2248,.F.);
#2788=ORIENTED_EDGE('',*,*,#2249,.F.);
#2789=ORIENTED_EDGE('',*,*,#2250,.T.);
#2790=ORIENTED_EDGE('',*,*,#2207,.T.);
#2791=ORIENTED_EDGE('',*,*,#2251,.T.);
#2792=ORIENTED_EDGE('',*,*,#2249,.T.);
#2793=ORIENTED_EDGE('',*,*,#2252,.F.);
#2794=ORIENTED_EDGE('',*,*,#2184,.T.);
#2795=ORIENTED_EDGE('',*,*,#2253,.F.);
#2796=ORIENTED_EDGE('',*,*,#2254,.F.);
#2797=ORIENTED_EDGE('',*,*,#2255,.T.);
#2798=ORIENTED_EDGE('',*,*,#2235,.T.);
#2799=ORIENTED_EDGE('',*,*,#2256,.T.);
#2800=ORIENTED_EDGE('',*,*,#2254,.T.);
#2801=ORIENTED_EDGE('',*,*,#2257,.F.);
#2802=ORIENTED_EDGE('',*,*,#2212,.T.);
#2803=ORIENTED_EDGE('',*,*,#2258,.F.);
#2804=ORIENTED_EDGE('',*,*,#2241,.F.);
#2805=ORIENTED_EDGE('',*,*,#2259,.T.);
#2806=ORIENTED_EDGE('',*,*,#2127,.T.);
#2807=ORIENTED_EDGE('',*,*,#2131,.T.);
#2808=ORIENTED_EDGE('',*,*,#2134,.T.);
#2809=ORIENTED_EDGE('',*,*,#2137,.T.);
#2810=ORIENTED_EDGE('',*,*,#2140,.T.);
#2811=ORIENTED_EDGE('',*,*,#2143,.T.);
#2812=ORIENTED_EDGE('',*,*,#2146,.T.);
#2813=ORIENTED_EDGE('',*,*,#2149,.T.);
#2814=ORIENTED_EDGE('',*,*,#2152,.T.);
#2815=ORIENTED_EDGE('',*,*,#2242,.T.);
#2816=ORIENTED_EDGE('',*,*,#2258,.T.);
#2817=ORIENTED_EDGE('',*,*,#2211,.T.);
#2818=ORIENTED_EDGE('',*,*,#2215,.T.);
#2819=ORIENTED_EDGE('',*,*,#2218,.T.);
#2820=ORIENTED_EDGE('',*,*,#2221,.T.);
#2821=ORIENTED_EDGE('',*,*,#2224,.T.);
#2822=ORIENTED_EDGE('',*,*,#2227,.T.);
#2823=ORIENTED_EDGE('',*,*,#2230,.T.);
#2824=ORIENTED_EDGE('',*,*,#2233,.T.);
#2825=ORIENTED_EDGE('',*,*,#2236,.T.);
#2826=ORIENTED_EDGE('',*,*,#2257,.T.);
#2827=ORIENTED_EDGE('',*,*,#2253,.T.);
#2828=ORIENTED_EDGE('',*,*,#2183,.T.);
#2829=ORIENTED_EDGE('',*,*,#2187,.T.);
#2830=ORIENTED_EDGE('',*,*,#2190,.T.);
#2831=ORIENTED_EDGE('',*,*,#2193,.T.);
#2832=ORIENTED_EDGE('',*,*,#2196,.T.);
#2833=ORIENTED_EDGE('',*,*,#2199,.T.);
#2834=ORIENTED_EDGE('',*,*,#2202,.T.);
#2835=ORIENTED_EDGE('',*,*,#2205,.T.);
#2836=ORIENTED_EDGE('',*,*,#2208,.T.);
#2837=ORIENTED_EDGE('',*,*,#2252,.T.);
#2838=ORIENTED_EDGE('',*,*,#2248,.T.);
#2839=ORIENTED_EDGE('',*,*,#2155,.T.);
#2840=ORIENTED_EDGE('',*,*,#2159,.T.);
#2841=ORIENTED_EDGE('',*,*,#2162,.T.);
#2842=ORIENTED_EDGE('',*,*,#2165,.T.);
#2843=ORIENTED_EDGE('',*,*,#2168,.T.);
#2844=ORIENTED_EDGE('',*,*,#2171,.T.);
#2845=ORIENTED_EDGE('',*,*,#2174,.T.);
#2846=ORIENTED_EDGE('',*,*,#2177,.T.);
#2847=ORIENTED_EDGE('',*,*,#2180,.T.);
#2848=ORIENTED_EDGE('',*,*,#2247,.T.);
#2849=ORIENTED_EDGE('',*,*,#2243,.T.);
#2850=ORIENTED_EDGE('',*,*,#2239,.T.);
#2851=ORIENTED_EDGE('',*,*,#2125,.T.);
#2852=ORIENTED_EDGE('',*,*,#2245,.F.);
#2853=ORIENTED_EDGE('',*,*,#2246,.F.);
#2854=ORIENTED_EDGE('',*,*,#2178,.T.);
#2855=ORIENTED_EDGE('',*,*,#2175,.T.);
#2856=ORIENTED_EDGE('',*,*,#2172,.T.);
#2857=ORIENTED_EDGE('',*,*,#2169,.T.);
#2858=ORIENTED_EDGE('',*,*,#2166,.T.);
#2859=ORIENTED_EDGE('',*,*,#2163,.T.);
#2860=ORIENTED_EDGE('',*,*,#2160,.T.);
#2861=ORIENTED_EDGE('',*,*,#2157,.T.);
#2862=ORIENTED_EDGE('',*,*,#2153,.T.);
#2863=ORIENTED_EDGE('',*,*,#2250,.F.);
#2864=ORIENTED_EDGE('',*,*,#2251,.F.);
#2865=ORIENTED_EDGE('',*,*,#2206,.T.);
#2866=ORIENTED_EDGE('',*,*,#2203,.T.);
#2867=ORIENTED_EDGE('',*,*,#2200,.T.);
#2868=ORIENTED_EDGE('',*,*,#2197,.T.);
#2869=ORIENTED_EDGE('',*,*,#2194,.T.);
#2870=ORIENTED_EDGE('',*,*,#2191,.T.);
#2871=ORIENTED_EDGE('',*,*,#2188,.T.);
#2872=ORIENTED_EDGE('',*,*,#2185,.T.);
#2873=ORIENTED_EDGE('',*,*,#2181,.T.);
#2874=ORIENTED_EDGE('',*,*,#2255,.F.);
#2875=ORIENTED_EDGE('',*,*,#2256,.F.);
#2876=ORIENTED_EDGE('',*,*,#2234,.T.);
#2877=ORIENTED_EDGE('',*,*,#2231,.T.);
#2878=ORIENTED_EDGE('',*,*,#2228,.T.);
#2879=ORIENTED_EDGE('',*,*,#2225,.T.);
#2880=ORIENTED_EDGE('',*,*,#2222,.T.);
#2881=ORIENTED_EDGE('',*,*,#2219,.T.);
#2882=ORIENTED_EDGE('',*,*,#2216,.T.);
#2883=ORIENTED_EDGE('',*,*,#2213,.T.);
#2884=ORIENTED_EDGE('',*,*,#2209,.T.);
#2885=ORIENTED_EDGE('',*,*,#2259,.F.);
#2886=ORIENTED_EDGE('',*,*,#2240,.F.);
#2887=ORIENTED_EDGE('',*,*,#2150,.T.);
#2888=ORIENTED_EDGE('',*,*,#2147,.T.);
#2889=ORIENTED_EDGE('',*,*,#2144,.T.);
#2890=ORIENTED_EDGE('',*,*,#2141,.T.);
#2891=ORIENTED_EDGE('',*,*,#2138,.T.);
#2892=ORIENTED_EDGE('',*,*,#2135,.T.);
#2893=ORIENTED_EDGE('',*,*,#2132,.T.);
#2894=ORIENTED_EDGE('',*,*,#2129,.T.);
#2895=ORIENTED_EDGE('',*,*,#2237,.T.);
#3558=CYLINDRICAL_SURFACE('',#4046,0.21);
#3600=ADVANCED_FACE('',(#531),#378,.F.);
#3601=ADVANCED_FACE('',(#532),#379,.F.);
#3602=ADVANCED_FACE('',(#533),#380,.F.);
#3603=ADVANCED_FACE('',(#534),#381,.F.);
#3604=ADVANCED_FACE('',(#535),#382,.F.);
#3605=ADVANCED_FACE('',(#536),#383,.F.);
#3606=ADVANCED_FACE('',(#537),#384,.F.);
#3607=ADVANCED_FACE('',(#538),#385,.F.);
#3608=ADVANCED_FACE('',(#539),#386,.F.);
#3609=ADVANCED_FACE('',(#540),#387,.F.);
#3610=ADVANCED_FACE('',(#541),#388,.F.);
#3611=ADVANCED_FACE('',(#542),#389,.F.);
#3612=ADVANCED_FACE('',(#543),#390,.F.);
#3613=ADVANCED_FACE('',(#544),#391,.F.);
#3614=ADVANCED_FACE('',(#545),#392,.F.);
#3615=ADVANCED_FACE('',(#546),#393,.F.);
#3616=ADVANCED_FACE('',(#547),#394,.F.);
#3617=ADVANCED_FACE('',(#548),#395,.F.);
#3618=ADVANCED_FACE('',(#549),#396,.F.);
#3619=ADVANCED_FACE('',(#550),#397,.F.);
#3620=ADVANCED_FACE('',(#551),#398,.F.);
#3621=ADVANCED_FACE('',(#552),#399,.F.);
#3622=ADVANCED_FACE('',(#553),#400,.F.);
#3623=ADVANCED_FACE('',(#554),#401,.F.);
#3624=ADVANCED_FACE('',(#555),#402,.F.);
#3625=ADVANCED_FACE('',(#556),#403,.F.);
#3626=ADVANCED_FACE('',(#557),#404,.F.);
#3627=ADVANCED_FACE('',(#558),#405,.F.);
#3628=ADVANCED_FACE('',(#559),#406,.F.);
#3629=ADVANCED_FACE('',(#560),#407,.F.);
#3630=ADVANCED_FACE('',(#561),#408,.F.);
#3631=ADVANCED_FACE('',(#562),#409,.F.);
#3632=ADVANCED_FACE('',(#563),#410,.F.);
#3633=ADVANCED_FACE('',(#564),#411,.F.);
#3634=ADVANCED_FACE('',(#565),#412,.F.);
#3635=ADVANCED_FACE('',(#566),#413,.F.);
#3636=ADVANCED_FACE('',(#567),#3558,.F.);
#3637=ADVANCED_FACE('',(#568),#414,.T.);
#3638=ADVANCED_FACE('',(#569),#415,.T.);
#3639=ADVANCED_FACE('',(#570),#416,.T.);
#3640=ADVANCED_FACE('',(#571),#417,.T.);
#3641=ADVANCED_FACE('',(#572),#418,.T.);
#3642=ADVANCED_FACE('',(#573),#419,.T.);
#3643=ADVANCED_FACE('',(#574),#420,.T.);
#3644=ADVANCED_FACE('',(#575),#421,.T.);
#3645=ADVANCED_FACE('',(#576,#329),#422,.T.);
#3646=ADVANCED_FACE('',(#577,#330),#423,.F.);
#3799=CLOSED_SHELL('',(#3600,#3601,#3602,#3603,#3604,#3605,#3606,#3607,
#3608,#3609,#3610,#3611,#3612,#3613,#3614,#3615,#3616,#3617,#3618,#3619,
#3620,#3621,#3622,#3623,#3624,#3625,#3626,#3627,#3628,#3629,#3630,#3631,
#3632,#3633,#3634,#3635,#3636,#3637,#3638,#3639,#3640,#3641,#3642,#3643,
#3644,#3645,#3646));
#4009=AXIS2_PLACEMENT_3D('',#5503,#4408,#4409);
#4010=AXIS2_PLACEMENT_3D('',#5504,#4410,#4411);
#4011=AXIS2_PLACEMENT_3D('',#5513,#4416,#4417);
#4012=AXIS2_PLACEMENT_3D('',#5519,#4421,#4422);
#4013=AXIS2_PLACEMENT_3D('',#5525,#4426,#4427);
#4014=AXIS2_PLACEMENT_3D('',#5531,#4431,#4432);
#4015=AXIS2_PLACEMENT_3D('',#5537,#4436,#4437);
#4016=AXIS2_PLACEMENT_3D('',#5543,#4441,#4442);
#4017=AXIS2_PLACEMENT_3D('',#5549,#4446,#4447);
#4018=AXIS2_PLACEMENT_3D('',#5555,#4451,#4452);
#4019=AXIS2_PLACEMENT_3D('',#5561,#4456,#4457);
#4020=AXIS2_PLACEMENT_3D('',#5570,#4462,#4463);
#4021=AXIS2_PLACEMENT_3D('',#5576,#4467,#4468);
#4022=AXIS2_PLACEMENT_3D('',#5582,#4472,#4473);
#4023=AXIS2_PLACEMENT_3D('',#5588,#4477,#4478);
#4024=AXIS2_PLACEMENT_3D('',#5594,#4482,#4483);
#4025=AXIS2_PLACEMENT_3D('',#5600,#4487,#4488);
#4026=AXIS2_PLACEMENT_3D('',#5606,#4492,#4493);
#4027=AXIS2_PLACEMENT_3D('',#5612,#4497,#4498);
#4028=AXIS2_PLACEMENT_3D('',#5618,#4502,#4503);
#4029=AXIS2_PLACEMENT_3D('',#5627,#4508,#4509);
#4030=AXIS2_PLACEMENT_3D('',#5633,#4513,#4514);
#4031=AXIS2_PLACEMENT_3D('',#5639,#4518,#4519);
#4032=AXIS2_PLACEMENT_3D('',#5645,#4523,#4524);
#4033=AXIS2_PLACEMENT_3D('',#5651,#4528,#4529);
#4034=AXIS2_PLACEMENT_3D('',#5657,#4533,#4534);
#4035=AXIS2_PLACEMENT_3D('',#5663,#4538,#4539);
#4036=AXIS2_PLACEMENT_3D('',#5669,#4543,#4544);
#4037=AXIS2_PLACEMENT_3D('',#5675,#4548,#4549);
#4038=AXIS2_PLACEMENT_3D('',#5684,#4554,#4555);
#4039=AXIS2_PLACEMENT_3D('',#5690,#4559,#4560);
#4040=AXIS2_PLACEMENT_3D('',#5696,#4564,#4565);
#4041=AXIS2_PLACEMENT_3D('',#5702,#4569,#4570);
#4042=AXIS2_PLACEMENT_3D('',#5708,#4574,#4575);
#4043=AXIS2_PLACEMENT_3D('',#5714,#4579,#4580);
#4044=AXIS2_PLACEMENT_3D('',#5720,#4584,#4585);
#4045=AXIS2_PLACEMENT_3D('',#5726,#4589,#4590);
#4046=AXIS2_PLACEMENT_3D('',#5732,#4594,#4595);
#4047=AXIS2_PLACEMENT_3D('',#5734,#4596,#4597);
#4048=AXIS2_PLACEMENT_3D('',#5737,#4599,#4600);
#4049=AXIS2_PLACEMENT_3D('',#5738,#4601,#4602);
#4050=AXIS2_PLACEMENT_3D('',#5744,#4606,#4607);
#4051=AXIS2_PLACEMENT_3D('',#5750,#4611,#4612);
#4052=AXIS2_PLACEMENT_3D('',#5753,#4615,#4616);
#4053=AXIS2_PLACEMENT_3D('',#5759,#4620,#4621);
#4054=AXIS2_PLACEMENT_3D('',#5762,#4624,#4625);
#4055=AXIS2_PLACEMENT_3D('',#5768,#4629,#4630);
#4056=AXIS2_PLACEMENT_3D('',#5771,#4633,#4634);
#4057=AXIS2_PLACEMENT_3D('',#5774,#4637,#4638);
#4058=AXIS2_PLACEMENT_3D('',#5775,#4639,#4640);
#4408=DIRECTION('axis',(0.,0.,1.));
#4409=DIRECTION('refdir',(1.,0.,0.));
#4410=DIRECTION('center_axis',(0.,0.,-1.));
#4411=DIRECTION('ref_axis',(0.,1.,0.));
#4412=DIRECTION('',(0.,1.,0.));
#4413=DIRECTION('',(1.,0.,0.));
#4414=DIRECTION('',(0.,-1.,0.));
#4415=DIRECTION('',(1.,0.,0.));
#4416=DIRECTION('center_axis',(0.,1.,-8.88178419700125E-16));
#4417=DIRECTION('ref_axis',(0.,8.88178419700125E-16,1.));
#4418=DIRECTION('',(0.,8.88178419700125E-16,1.));
#4419=DIRECTION('',(1.,0.,0.));
#4420=DIRECTION('',(0.,-8.88178419700125E-16,-1.));
#4421=DIRECTION('center_axis',(0.,-7.40148683083439E-16,-1.));
#4422=DIRECTION('ref_axis',(0.,1.,-7.40148683083439E-16));
#4423=DIRECTION('',(0.,1.,-7.40148683083439E-16));
#4424=DIRECTION('',(1.,0.,0.));
#4425=DIRECTION('',(0.,-1.,7.40148683083439E-16));
#4426=DIRECTION('center_axis',(0.,-0.707106781186547,-0.707106781186548));
#4427=DIRECTION('ref_axis',(0.,0.707106781186548,-0.707106781186547));
#4428=DIRECTION('',(0.,0.707106781186548,-0.707106781186547));
#4429=DIRECTION('',(1.,0.,0.));
#4430=DIRECTION('',(0.,-0.707106781186548,0.707106781186547));
#4431=DIRECTION('center_axis',(0.,-1.,2.77555756156289E-16));
#4432=DIRECTION('ref_axis',(0.,-2.77555756156289E-16,-1.));
#4433=DIRECTION('',(0.,-2.77555756156289E-16,-1.));
#4434=DIRECTION('',(1.,0.,0.));
#4435=DIRECTION('',(0.,2.77555756156289E-16,1.));
#4436=DIRECTION('center_axis',(0.,-0.707106781186547,0.707106781186548));
#4437=DIRECTION('ref_axis',(0.,-0.707106781186548,-0.707106781186547));
#4438=DIRECTION('',(0.,-0.707106781186548,-0.707106781186547));
#4439=DIRECTION('',(1.,0.,0.));
#4440=DIRECTION('',(0.,0.707106781186548,0.707106781186547));
#4441=DIRECTION('center_axis',(0.,7.40148683083438E-16,1.));
#4442=DIRECTION('ref_axis',(0.,-1.,7.40148683083438E-16));
#4443=DIRECTION('',(0.,-1.,7.40148683083438E-16));
#4444=DIRECTION('',(1.,0.,0.));
#4445=DIRECTION('',(0.,1.,-7.40148683083438E-16));
#4446=DIRECTION('center_axis',(0.,1.,-4.44089209850063E-16));
#4447=DIRECTION('ref_axis',(0.,4.44089209850063E-16,1.));
#4448=DIRECTION('',(0.,4.44089209850063E-16,1.));
#4449=DIRECTION('',(1.,0.,0.));
#4450=DIRECTION('',(0.,-4.44089209850063E-16,-1.));
#4451=DIRECTION('center_axis',(0.,2.41352831440251E-16,1.));
#4452=DIRECTION('ref_axis',(0.,-1.,2.41352831440251E-16));
#4453=DIRECTION('',(0.,-1.,2.41352831440251E-16));
#4454=DIRECTION('',(-1.,0.,0.));
#4455=DIRECTION('',(0.,1.,-2.41352831440251E-16));
#4456=DIRECTION('center_axis',(0.,-1.,2.41352831440251E-16));
#4457=DIRECTION('ref_axis',(0.,-2.41352831440251E-16,-1.));
#4458=DIRECTION('',(0.,-2.41352831440251E-16,-1.));
#4459=DIRECTION('',(1.,0.,0.));
#4460=DIRECTION('',(0.,2.41352831440251E-16,1.));
#4461=DIRECTION('',(1.,0.,0.));
#4462=DIRECTION('center_axis',(0.,0.,-1.));
#4463=DIRECTION('ref_axis',(0.,1.,0.));
#4464=DIRECTION('',(0.,1.,0.));
#4465=DIRECTION('',(1.,0.,0.));
#4466=DIRECTION('',(0.,-1.,0.));
#4467=DIRECTION('center_axis',(0.,-1.,0.));
#4468=DIRECTION('ref_axis',(0.,0.,-1.));
#4469=DIRECTION('',(0.,0.,-1.));
#4470=DIRECTION('',(1.,0.,0.));
#4471=DIRECTION('',(0.,0.,1.));
#4472=DIRECTION('center_axis',(0.,-0.707106781186547,0.707106781186548));
#4473=DIRECTION('ref_axis',(0.,-0.707106781186548,-0.707106781186547));
#4474=DIRECTION('',(0.,-0.707106781186548,-0.707106781186547));
#4475=DIRECTION('',(1.,0.,0.));
#4476=DIRECTION('',(0.,0.707106781186548,0.707106781186547));
#4477=DIRECTION('center_axis',(0.,0.,1.));
#4478=DIRECTION('ref_axis',(0.,-1.,0.));
#4479=DIRECTION('',(0.,-1.,0.));
#4480=DIRECTION('',(1.,0.,0.));
#4481=DIRECTION('',(0.,1.,0.));
#4482=DIRECTION('center_axis',(0.,0.707106781186548,0.707106781186547));
#4483=DIRECTION('ref_axis',(0.,-0.707106781186547,0.707106781186548));
#4484=DIRECTION('',(0.,-0.707106781186547,0.707106781186548));
#4485=DIRECTION('',(1.,0.,0.));
#4486=DIRECTION('',(0.,0.707106781186547,-0.707106781186548));
#4487=DIRECTION('center_axis',(0.,1.,0.));
#4488=DIRECTION('ref_axis',(0.,0.,1.));
#4489=DIRECTION('',(0.,0.,1.));
#4490=DIRECTION('',(1.,0.,0.));
#4491=DIRECTION('',(0.,0.,-1.));
#4492=DIRECTION('center_axis',(0.,0.,-1.));
#4493=DIRECTION('ref_axis',(0.,1.,0.));
#4494=DIRECTION('',(0.,1.,0.));
#4495=DIRECTION('',(1.,0.,0.));
#4496=DIRECTION('',(0.,-1.,0.));
#4497=DIRECTION('center_axis',(0.,1.,-2.41352831440251E-16));
#4498=DIRECTION('ref_axis',(0.,2.41352831440251E-16,1.));
#4499=DIRECTION('',(0.,2.41352831440251E-16,1.));
#4500=DIRECTION('',(-1.,0.,0.));
#4501=DIRECTION('',(0.,-2.41352831440251E-16,-1.));
#4502=DIRECTION('center_axis',(0.,0.,1.));
#4503=DIRECTION('ref_axis',(0.,-1.,0.));
#4504=DIRECTION('',(0.,-1.,0.));
#4505=DIRECTION('',(1.,0.,0.));
#4506=DIRECTION('',(0.,1.,0.));
#4507=DIRECTION('',(1.,0.,0.));
#4508=DIRECTION('center_axis',(0.,-1.,0.));
#4509=DIRECTION('ref_axis',(0.,0.,-1.));
#4510=DIRECTION('',(0.,0.,-1.));
#4511=DIRECTION('',(1.,0.,0.));
#4512=DIRECTION('',(0.,0.,1.));
#4513=DIRECTION('center_axis',(0.,0.,1.));
#4514=DIRECTION('ref_axis',(0.,-1.,0.));
#4515=DIRECTION('',(0.,-1.,0.));
#4516=DIRECTION('',(1.,0.,0.));
#4517=DIRECTION('',(0.,1.,0.));
#4518=DIRECTION('center_axis',(0.,0.707106781186548,0.707106781186548));
#4519=DIRECTION('ref_axis',(0.,-0.707106781186548,0.707106781186548));
#4520=DIRECTION('',(0.,-0.707106781186548,0.707106781186548));
#4521=DIRECTION('',(1.,0.,0.));
#4522=DIRECTION('',(0.,0.707106781186548,-0.707106781186548));
#4523=DIRECTION('center_axis',(0.,1.,0.));
#4524=DIRECTION('ref_axis',(0.,0.,1.));
#4525=DIRECTION('',(0.,0.,1.));
#4526=DIRECTION('',(1.,0.,0.));
#4527=DIRECTION('',(0.,0.,-1.));
#4528=DIRECTION('center_axis',(0.,0.707106781186548,-0.707106781186547));
#4529=DIRECTION('ref_axis',(0.,0.707106781186547,0.707106781186548));
#4530=DIRECTION('',(0.,0.707106781186547,0.707106781186548));
#4531=DIRECTION('',(1.,0.,0.));
#4532=DIRECTION('',(0.,-0.707106781186547,-0.707106781186548));
#4533=DIRECTION('center_axis',(0.,-7.40148683083438E-16,-1.));
#4534=DIRECTION('ref_axis',(0.,1.,-7.40148683083438E-16));
#4535=DIRECTION('',(0.,1.,-7.40148683083438E-16));
#4536=DIRECTION('',(1.,0.,0.));
#4537=DIRECTION('',(0.,-1.,7.40148683083438E-16));
#4538=DIRECTION('center_axis',(0.,-1.,0.));
#4539=DIRECTION('ref_axis',(0.,0.,-1.));
#4540=DIRECTION('',(0.,0.,-1.));
#4541=DIRECTION('',(1.,0.,0.));
#4542=DIRECTION('',(0.,0.,1.));
#4543=DIRECTION('center_axis',(0.,0.,-1.));
#4544=DIRECTION('ref_axis',(0.,1.,0.));
#4545=DIRECTION('',(0.,1.,0.));
#4546=DIRECTION('',(-1.,0.,0.));
#4547=DIRECTION('',(0.,-1.,0.));
#4548=DIRECTION('center_axis',(0.,1.,0.));
#4549=DIRECTION('ref_axis',(0.,0.,1.));
#4550=DIRECTION('',(0.,0.,1.));
#4551=DIRECTION('',(1.,0.,0.));
#4552=DIRECTION('',(0.,0.,-1.));
#4553=DIRECTION('',(1.,0.,0.));
#4554=DIRECTION('center_axis',(0.,0.,1.));
#4555=DIRECTION('ref_axis',(0.,-1.,0.));
#4556=DIRECTION('',(0.,-1.,0.));
#4557=DIRECTION('',(1.,0.,0.));
#4558=DIRECTION('',(0.,1.,0.));
#4559=DIRECTION('center_axis',(0.,1.,0.));
#4560=DIRECTION('ref_axis',(0.,0.,1.));
#4561=DIRECTION('',(0.,0.,1.));
#4562=DIRECTION('',(1.,0.,0.));
#4563=DIRECTION('',(0.,0.,-1.));
#4564=DIRECTION('center_axis',(0.,0.707106781186547,-0.707106781186548));
#4565=DIRECTION('ref_axis',(0.,0.707106781186548,0.707106781186547));
#4566=DIRECTION('',(0.,0.707106781186548,0.707106781186547));
#4567=DIRECTION('',(1.,0.,0.));
#4568=DIRECTION('',(0.,-0.707106781186548,-0.707106781186547));
#4569=DIRECTION('center_axis',(0.,0.,-1.));
#4570=DIRECTION('ref_axis',(0.,1.,0.));
#4571=DIRECTION('',(0.,1.,0.));
#4572=DIRECTION('',(1.,0.,0.));
#4573=DIRECTION('',(0.,-1.,0.));
#4574=DIRECTION('center_axis',(0.,-0.707106781186547,-0.707106781186548));
#4575=DIRECTION('ref_axis',(0.,0.707106781186548,-0.707106781186547));
#4576=DIRECTION('',(0.,0.707106781186548,-0.707106781186547));
#4577=DIRECTION('',(1.,0.,0.));
#4578=DIRECTION('',(0.,-0.707106781186548,0.707106781186547));
#4579=DIRECTION('center_axis',(0.,-1.,0.));
#4580=DIRECTION('ref_axis',(0.,0.,-1.));
#4581=DIRECTION('',(0.,0.,-1.));
#4582=DIRECTION('',(1.,0.,0.));
#4583=DIRECTION('',(0.,0.,1.));
#4584=DIRECTION('center_axis',(0.,0.,1.));
#4585=DIRECTION('ref_axis',(0.,-1.,0.));
#4586=DIRECTION('',(0.,-1.,0.));
#4587=DIRECTION('',(1.,0.,0.));
#4588=DIRECTION('',(0.,1.,0.));
#4589=DIRECTION('center_axis',(0.,-1.,0.));
#4590=DIRECTION('ref_axis',(0.,0.,-1.));
#4591=DIRECTION('',(0.,0.,-1.));
#4592=DIRECTION('',(-1.,0.,0.));
#4593=DIRECTION('',(0.,0.,1.));
#4594=DIRECTION('center_axis',(1.,0.,0.));
#4595=DIRECTION('ref_axis',(0.,0.,-1.));
#4596=DIRECTION('center_axis',(1.,0.,0.));
#4597=DIRECTION('ref_axis',(0.,0.,-1.));
#4598=DIRECTION('',(1.,0.,0.));
#4599=DIRECTION('center_axis',(-1.,0.,0.));
#4600=DIRECTION('ref_axis',(0.,0.,-1.));
#4601=DIRECTION('center_axis',(0.,1.,0.));
#4602=DIRECTION('ref_axis',(0.,0.,1.));
#4603=DIRECTION('',(0.,0.,1.));
#4604=DIRECTION('',(1.,0.,0.));
#4605=DIRECTION('',(0.,0.,1.));
#4606=DIRECTION('center_axis',(0.,1.,0.));
#4607=DIRECTION('ref_axis',(0.,0.,1.));
#4608=DIRECTION('',(0.,0.,1.));
#4609=DIRECTION('',(1.,0.,0.));
#4610=DIRECTION('',(0.,0.,1.));
#4611=DIRECTION('center_axis',(0.,0.,-1.));
#4612=DIRECTION('ref_axis',(0.,1.,0.));
#4613=DIRECTION('',(0.,1.,0.));
#4614=DIRECTION('',(0.,1.,0.));
#4615=DIRECTION('center_axis',(0.,0.,-1.));
#4616=DIRECTION('ref_axis',(0.,1.,0.));
#4617=DIRECTION('',(0.,1.,0.));
#4618=DIRECTION('',(1.,0.,0.));
#4619=DIRECTION('',(0.,1.,0.));
#4620=DIRECTION('center_axis',(0.,-1.,0.));
#4621=DIRECTION('ref_axis',(0.,0.,-1.));
#4622=DIRECTION('',(0.,0.,-1.));
#4623=DIRECTION('',(0.,0.,-1.));
#4624=DIRECTION('center_axis',(0.,-1.,0.));
#4625=DIRECTION('ref_axis',(0.,0.,-1.));
#4626=DIRECTION('',(0.,0.,-1.));
#4627=DIRECTION('',(1.,0.,0.));
#4628=DIRECTION('',(0.,0.,-1.));
#4629=DIRECTION('center_axis',(0.,0.,1.));
#4630=DIRECTION('ref_axis',(0.,-1.,0.));
#4631=DIRECTION('',(0.,-1.,0.));
#4632=DIRECTION('',(0.,-1.,0.));
#4633=DIRECTION('center_axis',(0.,0.,1.));
#4634=DIRECTION('ref_axis',(0.,-1.,0.));
#4635=DIRECTION('',(0.,-1.,0.));
#4636=DIRECTION('',(0.,-1.,0.));
#4637=DIRECTION('center_axis',(1.,0.,0.));
#4638=DIRECTION('ref_axis',(0.,0.,-1.));
#4639=DIRECTION('center_axis',(1.,0.,0.));
#4640=DIRECTION('ref_axis',(0.,0.,-1.));
#5503=CARTESIAN_POINT('',(0.,0.,0.));
#5504=CARTESIAN_POINT('Origin',(-0.1,0.82,-0.3));
#5505=CARTESIAN_POINT('',(0.,0.82,-0.3));
#5506=CARTESIAN_POINT('',(0.,1.,-0.3));
#5507=CARTESIAN_POINT('',(0.,0.41,-0.3));
#5508=CARTESIAN_POINT('',(30.,0.82,-0.3));
#5509=CARTESIAN_POINT('',(-0.1,0.82,-0.3));
#5510=CARTESIAN_POINT('',(30.,1.,-0.3));
#5511=CARTESIAN_POINT('',(30.,0.41,-0.3));
#5512=CARTESIAN_POINT('',(-0.05,1.,-0.3));
#5513=CARTESIAN_POINT('Origin',(-0.1,0.82,-0.55));
#5514=CARTESIAN_POINT('',(0.,0.82,-0.55));
#5515=CARTESIAN_POINT('',(0.,0.82,-0.275));
#5516=CARTESIAN_POINT('',(30.,0.82,-0.55));
#5517=CARTESIAN_POINT('',(-0.1,0.82,-0.55));
#5518=CARTESIAN_POINT('',(30.,0.82,-0.275));
#5519=CARTESIAN_POINT('Origin',(-0.1,0.67,-0.55));
#5520=CARTESIAN_POINT('',(0.,0.67,-0.55));
#5521=CARTESIAN_POINT('',(0.,0.335,-0.55));
#5522=CARTESIAN_POINT('',(30.,0.67,-0.55));
#5523=CARTESIAN_POINT('',(-0.1,0.67,-0.55));
#5524=CARTESIAN_POINT('',(30.,0.335,-0.55));
#5525=CARTESIAN_POINT('Origin',(-0.1,0.42,-0.3));
#5526=CARTESIAN_POINT('',(0.,0.42,-0.3));
#5527=CARTESIAN_POINT('',(0.,0.24,-0.12));
#5528=CARTESIAN_POINT('',(30.,0.42,-0.3));
#5529=CARTESIAN_POINT('',(-0.1,0.42,-0.3));
#5530=CARTESIAN_POINT('',(30.,0.24,-0.12));
#5531=CARTESIAN_POINT('Origin',(-0.1,0.42,0.3));
#5532=CARTESIAN_POINT('',(0.,0.42,0.3));
#5533=CARTESIAN_POINT('',(0.,0.42,0.15));
#5534=CARTESIAN_POINT('',(30.,0.42,0.3));
#5535=CARTESIAN_POINT('',(-0.1,0.42,0.3));
#5536=CARTESIAN_POINT('',(30.,0.42,0.15));
#5537=CARTESIAN_POINT('Origin',(-0.1,0.67,0.55));
#5538=CARTESIAN_POINT('',(0.,0.67,0.55));
#5539=CARTESIAN_POINT('',(6.93889390390723E-18,0.365,0.245));
#5540=CARTESIAN_POINT('',(30.,0.67,0.55));
#5541=CARTESIAN_POINT('',(-0.1,0.67,0.55));
#5542=CARTESIAN_POINT('',(30.,0.365,0.245));
#5543=CARTESIAN_POINT('Origin',(-0.1,0.82,0.55));
#5544=CARTESIAN_POINT('',(0.,0.82,0.55));
#5545=CARTESIAN_POINT('',(0.,0.41,0.55));
#5546=CARTESIAN_POINT('',(30.,0.82,0.55));
#5547=CARTESIAN_POINT('',(-0.1,0.82,0.55));
#5548=CARTESIAN_POINT('',(30.,0.41,0.55));
#5549=CARTESIAN_POINT('Origin',(-0.1,0.82,0.3));
#5550=CARTESIAN_POINT('',(0.,0.82,0.3));
#5551=CARTESIAN_POINT('',(0.,0.82,0.15));
#5552=CARTESIAN_POINT('',(30.,0.82,0.3));
#5553=CARTESIAN_POINT('',(-0.1,0.82,0.3));
#5554=CARTESIAN_POINT('',(30.,0.82,0.15));
#5555=CARTESIAN_POINT('Origin',(-0.1,1.05,0.3));
#5556=CARTESIAN_POINT('',(0.,1.,0.3));
#5557=CARTESIAN_POINT('',(0.,0.525,0.3));
#5558=CARTESIAN_POINT('',(30.,1.,0.3));
#5559=CARTESIAN_POINT('',(-0.05,1.,0.3));
#5560=CARTESIAN_POINT('',(30.,0.525,0.3));
#5561=CARTESIAN_POINT('Origin',(-0.1,-0.3,-0.82));
#5562=CARTESIAN_POINT('',(0.,-0.3,-0.82));
#5563=CARTESIAN_POINT('',(0.,-0.3,-1.));
#5564=CARTESIAN_POINT('',(0.,-0.3,-0.41));
#5565=CARTESIAN_POINT('',(30.,-0.3,-0.82));
#5566=CARTESIAN_POINT('',(-0.1,-0.3,-0.82));
#5567=CARTESIAN_POINT('',(30.,-0.3,-1.));
#5568=CARTESIAN_POINT('',(30.,-0.3,-0.41));
#5569=CARTESIAN_POINT('',(-0.05,-0.3,-1.));
#5570=CARTESIAN_POINT('Origin',(-0.1,-0.55,-0.82));
#5571=CARTESIAN_POINT('',(0.,-0.55,-0.82));
#5572=CARTESIAN_POINT('',(0.,-0.275,-0.82));
#5573=CARTESIAN_POINT('',(30.,-0.55,-0.82));
#5574=CARTESIAN_POINT('',(-0.1,-0.55,-0.82));
#5575=CARTESIAN_POINT('',(30.,-0.275,-0.82));
#5576=CARTESIAN_POINT('Origin',(-0.1,-0.55,-0.67));
#5577=CARTESIAN_POINT('',(0.,-0.55,-0.67));
#5578=CARTESIAN_POINT('',(0.,-0.55,-0.335));
#5579=CARTESIAN_POINT('',(30.,-0.55,-0.67));
#5580=CARTESIAN_POINT('',(-0.1,-0.55,-0.67));
#5581=CARTESIAN_POINT('',(30.,-0.55,-0.335));
#5582=CARTESIAN_POINT('Origin',(-0.1,-0.3,-0.42));
#5583=CARTESIAN_POINT('',(0.,-0.3,-0.42));
#5584=CARTESIAN_POINT('',(0.,-0.12,-0.24));
#5585=CARTESIAN_POINT('',(30.,-0.3,-0.42));
#5586=CARTESIAN_POINT('',(-0.1,-0.3,-0.42));
#5587=CARTESIAN_POINT('',(30.,-0.12,-0.24));
#5588=CARTESIAN_POINT('Origin',(-0.1,0.3,-0.42));
#5589=CARTESIAN_POINT('',(0.,0.3,-0.42));
#5590=CARTESIAN_POINT('',(0.,0.15,-0.42));
#5591=CARTESIAN_POINT('',(30.,0.3,-0.42));
#5592=CARTESIAN_POINT('',(-0.1,0.3,-0.42));
#5593=CARTESIAN_POINT('',(30.,0.15,-0.42));
#5594=CARTESIAN_POINT('Origin',(-0.1,0.55,-0.67));
#5595=CARTESIAN_POINT('',(0.,0.55,-0.67));
#5596=CARTESIAN_POINT('',(0.,0.245,-0.365));
#5597=CARTESIAN_POINT('',(30.,0.55,-0.67));
#5598=CARTESIAN_POINT('',(-0.1,0.55,-0.67));
#5599=CARTESIAN_POINT('',(30.,0.245,-0.365));
#5600=CARTESIAN_POINT('Origin',(-0.1,0.55,-0.82));
#5601=CARTESIAN_POINT('',(0.,0.55,-0.82));
#5602=CARTESIAN_POINT('',(0.,0.55,-0.41));
#5603=CARTESIAN_POINT('',(30.,0.55,-0.82));
#5604=CARTESIAN_POINT('',(-0.1,0.55,-0.82));
#5605=CARTESIAN_POINT('',(30.,0.55,-0.41));
#5606=CARTESIAN_POINT('Origin',(-0.1,0.3,-0.82));
#5607=CARTESIAN_POINT('',(0.,0.3,-0.82));
#5608=CARTESIAN_POINT('',(0.,0.15,-0.82));
#5609=CARTESIAN_POINT('',(30.,0.3,-0.82));
#5610=CARTESIAN_POINT('',(-0.1,0.3,-0.82));
#5611=CARTESIAN_POINT('',(30.,0.15,-0.82));
#5612=CARTESIAN_POINT('Origin',(-0.1,0.3,-1.05));
#5613=CARTESIAN_POINT('',(0.,0.3,-1.));
#5614=CARTESIAN_POINT('',(0.,0.3,-0.525));
#5615=CARTESIAN_POINT('',(30.,0.3,-1.));
#5616=CARTESIAN_POINT('',(-0.05,0.3,-1.));
#5617=CARTESIAN_POINT('',(30.,0.3,-0.525));
#5618=CARTESIAN_POINT('Origin',(-0.1,-0.82,0.3));
#5619=CARTESIAN_POINT('',(0.,-0.82,0.3));
#5620=CARTESIAN_POINT('',(0.,-1.,0.3));
#5621=CARTESIAN_POINT('',(0.,-0.41,0.3));
#5622=CARTESIAN_POINT('',(30.,-0.82,0.3));
#5623=CARTESIAN_POINT('',(-0.1,-0.82,0.3));
#5624=CARTESIAN_POINT('',(30.,-1.,0.3));
#5625=CARTESIAN_POINT('',(30.,-0.41,0.3));
#5626=CARTESIAN_POINT('',(-0.05,-1.,0.3));
#5627=CARTESIAN_POINT('Origin',(-0.1,-0.82,0.55));
#5628=CARTESIAN_POINT('',(0.,-0.82,0.55));
#5629=CARTESIAN_POINT('',(0.,-0.82,0.275));
#5630=CARTESIAN_POINT('',(30.,-0.82,0.55));
#5631=CARTESIAN_POINT('',(-0.1,-0.82,0.55));
#5632=CARTESIAN_POINT('',(30.,-0.82,0.275));
#5633=CARTESIAN_POINT('Origin',(-0.1,-0.67,0.55));
#5634=CARTESIAN_POINT('',(0.,-0.67,0.55));
#5635=CARTESIAN_POINT('',(0.,-0.335,0.55));
#5636=CARTESIAN_POINT('',(30.,-0.67,0.55));
#5637=CARTESIAN_POINT('',(-0.1,-0.67,0.55));
#5638=CARTESIAN_POINT('',(30.,-0.335,0.55));
#5639=CARTESIAN_POINT('Origin',(-0.1,-0.42,0.3));
#5640=CARTESIAN_POINT('',(0.,-0.42,0.3));
#5641=CARTESIAN_POINT('',(-6.93889390390723E-18,-0.24,0.12));
#5642=CARTESIAN_POINT('',(30.,-0.42,0.3));
#5643=CARTESIAN_POINT('',(-0.1,-0.42,0.3));
#5644=CARTESIAN_POINT('',(30.,-0.24,0.12));
#5645=CARTESIAN_POINT('Origin',(-0.1,-0.42,-0.3));
#5646=CARTESIAN_POINT('',(0.,-0.42,-0.3));
#5647=CARTESIAN_POINT('',(0.,-0.42,-0.15));
#5648=CARTESIAN_POINT('',(30.,-0.42,-0.3));
#5649=CARTESIAN_POINT('',(-0.1,-0.42,-0.3));
#5650=CARTESIAN_POINT('',(30.,-0.42,-0.15));
#5651=CARTESIAN_POINT('Origin',(-0.1,-0.67,-0.55));
#5652=CARTESIAN_POINT('',(0.,-0.67,-0.55));
#5653=CARTESIAN_POINT('',(0.,-0.365,-0.245));
#5654=CARTESIAN_POINT('',(30.,-0.67,-0.55));
#5655=CARTESIAN_POINT('',(-0.1,-0.67,-0.55));
#5656=CARTESIAN_POINT('',(30.,-0.365,-0.245));
#5657=CARTESIAN_POINT('Origin',(-0.1,-0.82,-0.55));
#5658=CARTESIAN_POINT('',(0.,-0.82,-0.55));
#5659=CARTESIAN_POINT('',(0.,-0.41,-0.55));
#5660=CARTESIAN_POINT('',(30.,-0.82,-0.55));
#5661=CARTESIAN_POINT('',(-0.1,-0.82,-0.55));
#5662=CARTESIAN_POINT('',(30.,-0.41,-0.55));
#5663=CARTESIAN_POINT('Origin',(-0.1,-0.82,-0.3));
#5664=CARTESIAN_POINT('',(0.,-0.82,-0.3));
#5665=CARTESIAN_POINT('',(0.,-0.82,-0.15));
#5666=CARTESIAN_POINT('',(30.,-0.82,-0.3));
#5667=CARTESIAN_POINT('',(-0.1,-0.82,-0.3));
#5668=CARTESIAN_POINT('',(30.,-0.82,-0.15));
#5669=CARTESIAN_POINT('Origin',(-0.1,-1.05,-0.3));
#5670=CARTESIAN_POINT('',(0.,-1.,-0.3));
#5671=CARTESIAN_POINT('',(0.,-0.525,-0.3));
#5672=CARTESIAN_POINT('',(30.,-1.,-0.3));
#5673=CARTESIAN_POINT('',(-0.05,-1.,-0.3));
#5674=CARTESIAN_POINT('',(30.,-0.525,-0.3));
#5675=CARTESIAN_POINT('Origin',(-0.1,0.3,0.82));
#5676=CARTESIAN_POINT('',(0.,0.3,0.82));
#5677=CARTESIAN_POINT('',(0.,0.3,1.));
#5678=CARTESIAN_POINT('',(0.,0.3,0.41));
#5679=CARTESIAN_POINT('',(30.,0.3,0.82));
#5680=CARTESIAN_POINT('',(-0.1,0.3,0.82));
#5681=CARTESIAN_POINT('',(30.,0.3,1.));
#5682=CARTESIAN_POINT('',(30.,0.3,0.41));
#5683=CARTESIAN_POINT('',(-0.05,0.3,1.));
#5684=CARTESIAN_POINT('Origin',(-0.1,0.55,0.82));
#5685=CARTESIAN_POINT('',(0.,0.55,0.82));
#5686=CARTESIAN_POINT('',(0.,0.275,0.82));
#5687=CARTESIAN_POINT('',(30.,0.55,0.82));
#5688=CARTESIAN_POINT('',(-0.1,0.55,0.82));
#5689=CARTESIAN_POINT('',(30.,0.275,0.82));
#5690=CARTESIAN_POINT('Origin',(-0.1,0.55,0.67));
#5691=CARTESIAN_POINT('',(0.,0.55,0.67));
#5692=CARTESIAN_POINT('',(0.,0.55,0.335));
#5693=CARTESIAN_POINT('',(30.,0.55,0.67));
#5694=CARTESIAN_POINT('',(-0.1,0.55,0.67));
#5695=CARTESIAN_POINT('',(30.,0.55,0.335));
#5696=CARTESIAN_POINT('Origin',(-0.1,0.3,0.42));
#5697=CARTESIAN_POINT('',(0.,0.3,0.42));
#5698=CARTESIAN_POINT('',(6.93889390390723E-18,0.12,0.24));
#5699=CARTESIAN_POINT('',(30.,0.3,0.42));
#5700=CARTESIAN_POINT('',(-0.1,0.3,0.42));
#5701=CARTESIAN_POINT('',(30.,0.12,0.24));
#5702=CARTESIAN_POINT('Origin',(-0.1,-0.3,0.42));
#5703=CARTESIAN_POINT('',(0.,-0.3,0.42));
#5704=CARTESIAN_POINT('',(0.,-0.15,0.42));
#5705=CARTESIAN_POINT('',(30.,-0.3,0.42));
#5706=CARTESIAN_POINT('',(-0.1,-0.3,0.42));
#5707=CARTESIAN_POINT('',(30.,-0.15,0.42));
#5708=CARTESIAN_POINT('Origin',(-0.1,-0.55,0.67));
#5709=CARTESIAN_POINT('',(0.,-0.55,0.67));
#5710=CARTESIAN_POINT('',(6.93889390390723E-18,-0.245,0.365));
#5711=CARTESIAN_POINT('',(30.,-0.55,0.67));
#5712=CARTESIAN_POINT('',(-0.1,-0.55,0.67));
#5713=CARTESIAN_POINT('',(30.,-0.245,0.365));
#5714=CARTESIAN_POINT('Origin',(-0.1,-0.55,0.82));
#5715=CARTESIAN_POINT('',(0.,-0.55,0.82));
#5716=CARTESIAN_POINT('',(0.,-0.55,0.41));
#5717=CARTESIAN_POINT('',(30.,-0.55,0.82));
#5718=CARTESIAN_POINT('',(-0.1,-0.55,0.82));
#5719=CARTESIAN_POINT('',(30.,-0.55,0.41));
#5720=CARTESIAN_POINT('Origin',(-0.1,-0.3,0.82));
#5721=CARTESIAN_POINT('',(0.,-0.3,0.82));
#5722=CARTESIAN_POINT('',(0.,-0.15,0.82));
#5723=CARTESIAN_POINT('',(30.,-0.3,0.82));
#5724=CARTESIAN_POINT('',(-0.1,-0.3,0.82));
#5725=CARTESIAN_POINT('',(30.,-0.15,0.82));
#5726=CARTESIAN_POINT('Origin',(-0.1,-0.3,1.05));
#5727=CARTESIAN_POINT('',(0.,-0.3,1.));
#5728=CARTESIAN_POINT('',(0.,-0.3,0.525));
#5729=CARTESIAN_POINT('',(30.,-0.3,1.));
#5730=CARTESIAN_POINT('',(-0.05,-0.3,1.));
#5731=CARTESIAN_POINT('',(30.,-0.3,0.525));
#5732=CARTESIAN_POINT('Origin',(-0.1,0.,0.));
#5733=CARTESIAN_POINT('',(0.,-2.57175827820944E-17,0.21));
#5734=CARTESIAN_POINT('Origin',(0.,0.,0.));
#5735=CARTESIAN_POINT('',(30.,2.57175827820944E-17,0.21));
#5736=CARTESIAN_POINT('',(-0.1,-2.57175827820944E-17,0.21));
#5737=CARTESIAN_POINT('Origin',(30.,0.,0.));
#5738=CARTESIAN_POINT('Origin',(0.,1.,-1.));
#5739=CARTESIAN_POINT('',(0.,1.,1.));
#5740=CARTESIAN_POINT('',(0.,1.,-1.));
#5741=CARTESIAN_POINT('',(30.,1.,1.));
#5742=CARTESIAN_POINT('',(0.,1.,1.));
#5743=CARTESIAN_POINT('',(30.,1.,-1.));
#5744=CARTESIAN_POINT('Origin',(0.,1.,-1.));
#5745=CARTESIAN_POINT('',(30.,1.,-1.));
#5746=CARTESIAN_POINT('',(30.,1.,-1.));
#5747=CARTESIAN_POINT('',(0.,1.,-1.));
#5748=CARTESIAN_POINT('',(0.,1.,-1.));
#5749=CARTESIAN_POINT('',(0.,1.,-1.));
#5750=CARTESIAN_POINT('Origin',(0.,-1.,-1.));
#5751=CARTESIAN_POINT('',(0.,-1.,-1.));
#5752=CARTESIAN_POINT('',(30.,-1.,-1.));
#5753=CARTESIAN_POINT('Origin',(0.,-1.,-1.));
#5754=CARTESIAN_POINT('',(30.,-1.,-1.));
#5755=CARTESIAN_POINT('',(30.,-1.,-1.));
#5756=CARTESIAN_POINT('',(0.,-1.,-1.));
#5757=CARTESIAN_POINT('',(0.,-1.,-1.));
#5758=CARTESIAN_POINT('',(0.,-1.,-1.));
#5759=CARTESIAN_POINT('Origin',(0.,-1.,1.));
#5760=CARTESIAN_POINT('',(0.,-1.,1.));
#5761=CARTESIAN_POINT('',(30.,-1.,1.));
#5762=CARTESIAN_POINT('Origin',(0.,-1.,1.));
#5763=CARTESIAN_POINT('',(30.,-1.,1.));
#5764=CARTESIAN_POINT('',(30.,-1.,1.));
#5765=CARTESIAN_POINT('',(0.,-1.,1.));
#5766=CARTESIAN_POINT('',(0.,-1.,1.));
#5767=CARTESIAN_POINT('',(0.,-1.,1.));
#5768=CARTESIAN_POINT('Origin',(0.,1.,1.));
#5769=CARTESIAN_POINT('',(0.,1.,1.));
#5770=CARTESIAN_POINT('',(30.,1.,1.));
#5771=CARTESIAN_POINT('Origin',(0.,1.,1.));
#5772=CARTESIAN_POINT('',(30.,1.,1.));
#5773=CARTESIAN_POINT('',(0.,1.,1.));
#5774=CARTESIAN_POINT('Origin',(30.,0.,0.));
#5775=CARTESIAN_POINT('Origin',(0.,0.,0.));
#6705=UNCERTAINTY_MEASURE_WITH_UNIT(LENGTH_MEASURE(0.001),#6744,
'DISTANCE_ACCURACY_VALUE',
'Maximum model space distance between geometric entities at asserted c
onnectivities');
#6722=UNCERTAINTY_MEASURE_WITH_UNIT(LENGTH_MEASURE(0.001),#6744,
'DISTANCE_ACCURACY_VALUE',
'Maximum model space distance between geometric entities at asserted c
onnectivities');
#6726=(
GEOMETRIC_REPRESENTATION_CONTEXT(3)
GLOBAL_UNCERTAINTY_ASSIGNED_CONTEXT((#6705))
GLOBAL_UNIT_ASSIGNED_CONTEXT((#6744,#6746,#6747))
REPRESENTATION_CONTEXT('','3D')
);
#6743=(
GEOMETRIC_REPRESENTATION_CONTEXT(3)
GLOBAL_UNCERTAINTY_ASSIGNED_CONTEXT((#6722))
GLOBAL_UNIT_ASSIGNED_CONTEXT((#6744,#6746,#6747))
REPRESENTATION_CONTEXT('','3D')
);
#6744=(
LENGTH_UNIT()
NAMED_UNIT(*)
SI_UNIT(.CENTI.,.METRE.)
);
#6746=(
NAMED_UNIT(*)
PLANE_ANGLE_UNIT()
SI_UNIT($,.RADIAN.)
);
#6747=(
NAMED_UNIT(*)
SI_UNIT($,.STERADIAN.)
SOLID_ANGLE_UNIT()
);
#6751=SHAPE_DEFINITION_REPRESENTATION(#6771,#6840);
#6771=PRODUCT_DEFINITION_SHAPE('',$,#6861);
#6840=SHAPE_REPRESENTATION('',(#4009),#6726);
#6857=PRODUCT_DEFINITION_CONTEXT('part definition',#6919,'design');
#6861=PRODUCT_DEFINITION('Slotted Extrusion - 20 x 20 x 300 mm',
'Slotted Extrusion - 20 x 20 x 300 mm',#6881,#6857);
#6881=PRODUCT_DEFINITION_FORMATION('',$,#6924);
#6919=APPLICATION_CONTEXT(
'Core Data for Automotive Mechanical Design Process');
#6920=PRODUCT_CONTEXT('part definition',#6919,'mechanical');
#6924=PRODUCT('Slotted Extrusion - 20 x 20 x 300 mm',
'Slotted Extrusion - 20 x 20 x 300 mm',
'Slotted Extrusion - 20 x 20 x 300 mm',(#6920));
#7011=COLOUR_RGB('Off White',0.89,0.88,0.83);
#7012=FILL_AREA_STYLE_COLOUR('',#7011);
#7013=FILL_AREA_STYLE('',(#7012));
#7014=SURFACE_STYLE_FILL_AREA(#7013);
#7015=SURFACE_SIDE_STYLE('',(#7014));
#7016=SURFACE_STYLE_USAGE(.BOTH.,#7015);
#7017=PRESENTATION_STYLE_ASSIGNMENT((#7016));
ENDSEC;
END-ISO-10303-21;
